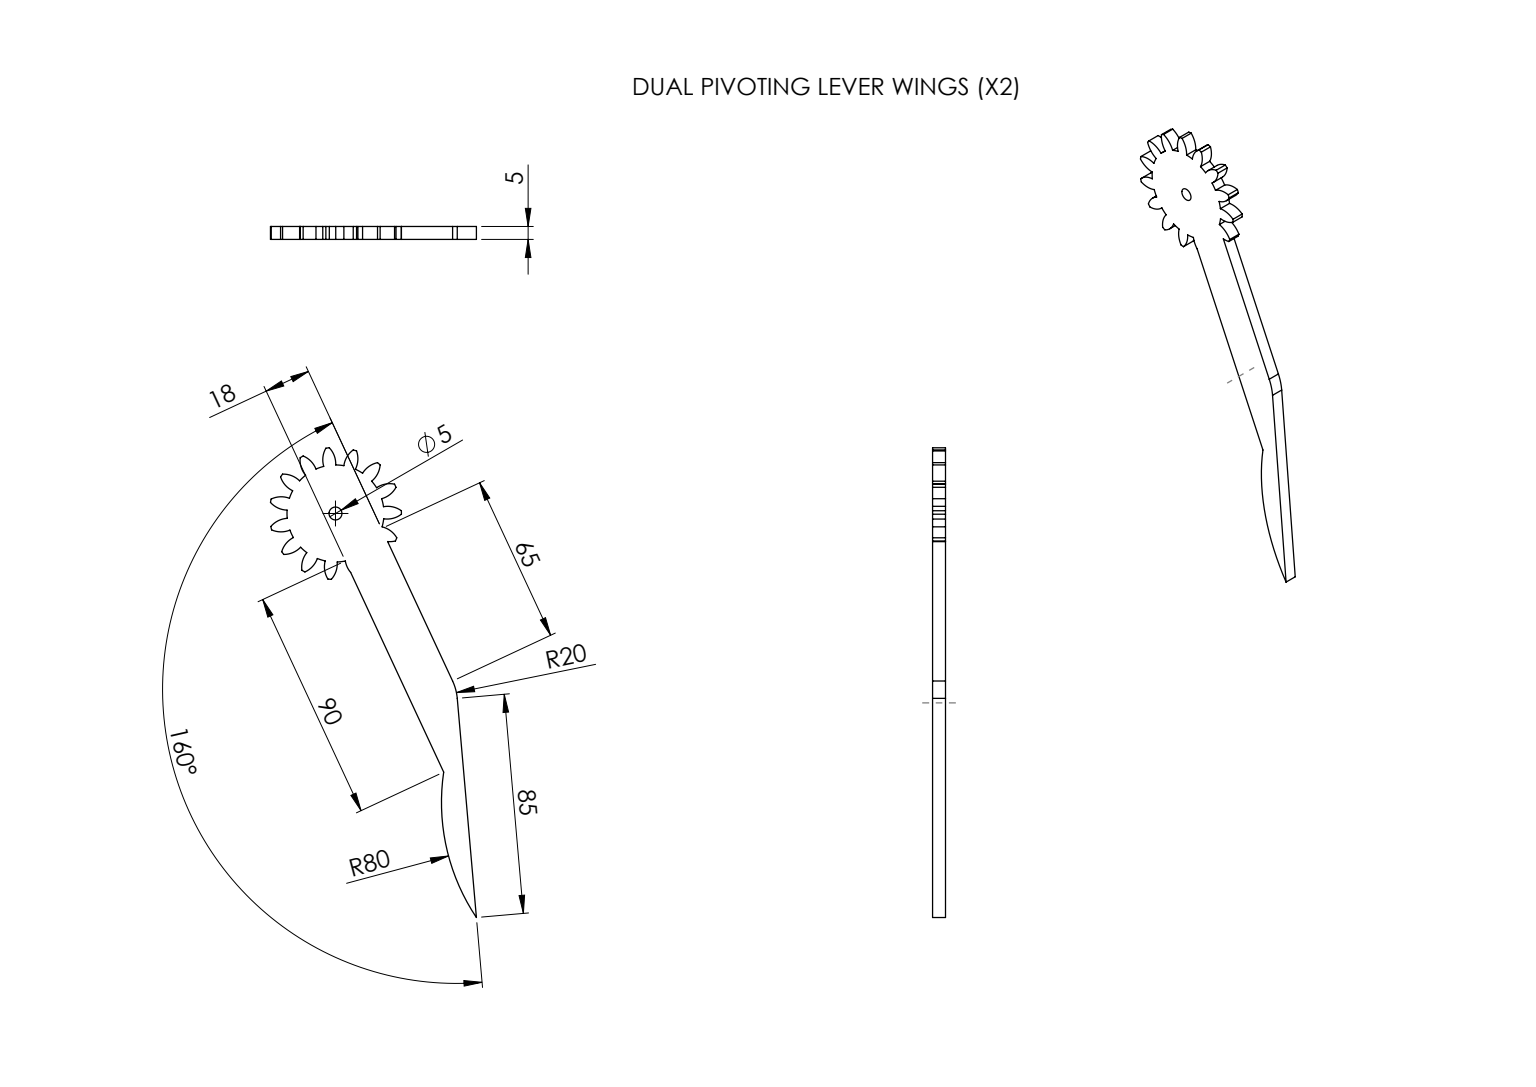
ISO-10303-21;
HEADER;
FILE_DESCRIPTION (('STEP AP214'),
    '1' );
FILE_NAME ('Dual Pivoting Lever Wings (x2).step',
    '2026-10-08T14:03:35',
    ( '' ),
    ( '' ),
    'SwSTEP 2.0',
    'SolidWorks 2026',
    '' );
FILE_SCHEMA (( 'AUTOMOTIVE_DESIGN' ));
ENDSEC;

DATA;
#2=ORIENTED_EDGE ( 'NONE', *, *, #10289, .F. ) ;
#4=VECTOR ( 'NONE', #10867, 1000.000000000000000 ) ;
#6=DIRECTION ( 'NONE',  ( 0.9960067511297464593, -0.08927794634716622324, 3.401418580343279473E-17 ) ) ;
#13=CARTESIAN_POINT ( 'NONE',  ( 34.99999999999958789, 1.104930248025249758E-13, -2.499999999999999112 ) ) ;
#17=EDGE_CURVE ( 'NONE', #9929, #10530, #4223, .T. ) ;
#25=EDGE_LOOP ( 'NONE', ( #11281, #8827, #8911, #8959 ) ) ;
#34=DIRECTION ( 'NONE',  ( 0.9960067511297463483, -0.08927794634716618161, 4.818676322152979407E-17 ) ) ;
#45=AXIS2_PLACEMENT_3D ( 'NONE', #8376, #5215, #8445 ) ;
#48=ORIENTED_EDGE ( 'NONE', *, *, #13831, .T. ) ;
#51=DIRECTION ( 'NONE',  ( 0.9960067511297463483, -0.08927794634716618161, 4.818676322152979407E-17 ) ) ;
#66=CARTESIAN_POINT ( 'NONE',  ( 34.99999999999958789, 1.104930248025249758E-13, -2.499999999999999112 ) ) ;
#68=DIRECTION ( 'NONE',  ( -6.158143864569485777E-17, -2.736152283717910599E-16, 1.000000000000000000 ) ) ;
#76=AXIS2_PLACEMENT_3D ( 'NONE', #13638, #11239, #6171 ) ;
#85=ORIENTED_EDGE ( 'NONE', *, *, #10554, .F. ) ;
#86=AXIS2_PLACEMENT_3D ( 'NONE', #6886, #3650, #3573 ) ;
#87=AXIS2_PLACEMENT_3D ( 'NONE', #13479, #2566, #7966 ) ;
#88=ADVANCED_FACE ( 'NONE', ( #12662 ), #10538, .T. ) ;
#89=DIRECTION ( 'NONE',  ( 6.158143864569485777E-17, 2.736152283717910599E-16, -1.000000000000000000 ) ) ;
#90=EDGE_CURVE ( 'NONE', #3108, #8314, #5574, .T. ) ;
#92=DIRECTION ( 'NONE',  ( -0.8735848310779960046, 0.4866719047884612293, 9.637352644305955116E-17 ) ) ;
#95=CARTESIAN_POINT ( 'NONE',  ( 21.12690199240172007, 12.61198448588842425, -2.499999999999996447 ) ) ;
#101=EDGE_CURVE ( 'NONE', #11832, #6555, #12065, .T. ) ;
#109=CARTESIAN_POINT ( 'NONE',  ( 43.14708730495711819, 24.16350488746832781, 2.500000000000007105 ) ) ;
#116=ORIENTED_EDGE ( 'NONE', *, *, #6600, .T. ) ;
#124=EDGE_CURVE ( 'NONE', #4194, #10453, #1869, .T. ) ;
#127=CYLINDRICAL_SURFACE ( 'NONE', #2611, 18.74900000001875000 ) ;
#128=CYLINDRICAL_SURFACE ( 'NONE', #1187, 18.74900000001875000 ) ;
#130=AXIS2_PLACEMENT_3D ( 'NONE', #4348, #7713, #2181 ) ;
#132=AXIS2_PLACEMENT_3D ( 'NONE', #2558, #4657, #7593 ) ;
#136=ORIENTED_EDGE ( 'NONE', *, *, #744, .F. ) ;
#153=CARTESIAN_POINT ( 'NONE',  ( 43.29712336220986657, 19.44704974301885159, -2.499999999999993783 ) ) ;
#155=( LENGTH_UNIT ( ) NAMED_UNIT ( * ) SI_UNIT ( .MILLI., .METRE. ) );
#157=DIRECTION ( 'NONE',  ( -0.6001121574638169642, 0.7999158696163758409, 1.927470528861191270E-16 ) ) ;
#160=CYLINDRICAL_SURFACE ( 'NONE', #3931, 25.50000000002549783 ) ;
#161=ORIENTED_EDGE ( 'NONE', *, *, #4188, .T. ) ;
#163=ORIENTED_EDGE ( 'NONE', *, *, #556, .F. ) ;
#167=ORIENTED_EDGE ( 'NONE', *, *, #10705, .F. ) ;
#168=CYLINDRICAL_SURFACE ( 'NONE', #12862, 25.50000000002549783 ) ;
#170=DIRECTION ( 'NONE',  ( -6.158143864569485777E-17, -2.736152283717910599E-16, 1.000000000000000000 ) ) ;
#172=CYLINDRICAL_SURFACE ( 'NONE', #13260, 80.00000000000001421 ) ;
#175=CARTESIAN_POINT ( 'NONE',  ( 53.63671053572210923, -2.048907369402451106, 2.500000000000000444 ) ) ;
#182=VERTEX_POINT ( 'NONE', #256 ) ;
#186=CARTESIAN_POINT ( 'NONE',  ( 41.86252833142972918, 24.55922850786694056, 2.500000000000007105 ) ) ;
#189=DIRECTION ( 'NONE',  ( -6.158143864569485777E-17, -2.736152283717910599E-16, 1.000000000000000000 ) ) ;
#197=ADVANCED_FACE ( 'NONE', ( #5497 ), #1357, .T. ) ;
#203=CARTESIAN_POINT ( 'NONE',  ( 80.29381926039658879, -64.72749139719506672, -2.500000000000000000 ) ) ;
#209=EDGE_LOOP ( 'NONE', ( #5485, #10650, #4189, #10104 ) ) ;
#216=ORIENTED_EDGE ( 'NONE', *, *, #1663, .T. ) ;
#220=DIRECTION ( 'NONE',  ( 0.1928999275155749149, 0.9812184353977894125, 2.775705599192072226E-16 ) ) ;
#222=DIRECTION ( 'NONE',  ( 6.158143864569485777E-17, 2.736152283717910599E-16, -1.000000000000000000 ) ) ;
#239=CIRCLE ( 'NONE', #906, 9.000000000008999024 ) ;
#242=ORIENTED_EDGE ( 'NONE', *, *, #7205, .T. ) ;
#254=CARTESIAN_POINT ( 'NONE',  ( 51.25836974494252019, 19.64472991003004054, 6.505213034913026604E-15 ) ) ;
#256=CARTESIAN_POINT ( 'NONE',  ( 23.90723890023449627, -15.11541108221136476, -2.500000000000003553 ) ) ;
#279=ORIENTED_EDGE ( 'NONE', *, *, #778, .T. ) ;
#288=FILL_AREA_STYLE_COLOUR ( '', #11871 ) ;
#290=DIRECTION ( 'NONE',  ( 0.000000000000000000, 0.000000000000000000, -1.000000000000000000 ) ) ;
#294=ORIENTED_EDGE ( 'NONE', *, *, #6674, .T. ) ;
#314=ORIENTED_EDGE ( 'NONE', *, *, #9696, .T. ) ;
#315=ORIENTED_EDGE ( 'NONE', *, *, #6674, .F. ) ;
#317=DIRECTION ( 'NONE',  ( -6.158143864569485777E-17, -2.736152283717910599E-16, 1.000000000000000000 ) ) ;
#319=CARTESIAN_POINT ( 'NONE',  ( 52.26118412238654543, 18.64354822589355365, 2.500000000000006217 ) ) ;
#321=EDGE_LOOP ( 'NONE', ( #4799, #6179, #1264, #10017 ) ) ;
#335=CARTESIAN_POINT ( 'NONE',  ( 14.79219767565757770, 6.218900627562692129, -2.499999999999999112 ) ) ;
#339=CIRCLE ( 'NONE', #9953, 18.74900000001874645 ) ;
#343=ORIENTED_EDGE ( 'NONE', *, *, #10693, .T. ) ;
#344=CARTESIAN_POINT ( 'NONE',  ( 22.31663499682298735, 16.91633092580596198, -2.499999999999995559 ) ) ;
#352=EDGE_CURVE ( 'NONE', #2949, #3802, #8059, .T. ) ;
#353=ORIENTED_EDGE ( 'NONE', *, *, #1966, .F. ) ;
#358=EDGE_LOOP ( 'NONE', ( #9572, #5128, #4628, #12509 ) ) ;
#361=CARTESIAN_POINT ( 'NONE',  ( 89.49979561504950709, -156.1132911148542917, 2.500000000000000000 ) ) ;
#363=DIRECTION ( 'NONE',  ( -6.158143864569485777E-17, -2.736152283717910599E-16, 1.000000000000000000 ) ) ;
#378=DIRECTION ( 'NONE',  ( -6.158143864569485777E-17, -2.736152283717910599E-16, 1.000000000000000000 ) ) ;
#382=DIRECTION ( 'NONE',  ( 1.000000000000000000, 0.000000000000000000, 0.000000000000000000 ) ) ;
#389=CARTESIAN_POINT ( 'NONE',  ( 37.49001687782395464, -0.2231948658678056807, 2.500000000000000000 ) ) ;
#390=DIRECTION ( 'NONE',  ( 0.9960067511297464593, -0.08927794634716622324, 3.401418580343279473E-17 ) ) ;
#391=CARTESIAN_POINT ( 'NONE',  ( 22.49448184590488609, 22.22300645049885048, 5.637851296924623057E-15 ) ) ;
#393=ORIENTED_EDGE ( 'NONE', *, *, #4024, .T. ) ;
#403=DIRECTION ( 'NONE',  ( 0.000000000000000000, 0.000000000000000000, 1.000000000000000000 ) ) ;
#404=CARTESIAN_POINT ( 'NONE',  ( 34.99999999999958789, 1.104930248025249758E-13, -2.499999999999999112 ) ) ;
#412=DIRECTION ( 'NONE',  ( 0.9960067511297463483, -0.08927794634716620936, 4.818676322152979407E-17 ) ) ;
#419=PLANE ( 'NONE',  #6579 ) ;
#420=VERTEX_POINT ( 'NONE', #8511 ) ;
#425=VERTEX_POINT ( 'NONE', #1859 ) ;
#434=DIRECTION ( 'NONE',  ( 0.9960067511297463483, -0.08927794634716620936, 4.626175998653454121E-17 ) ) ;
#439=ORIENTED_EDGE ( 'NONE', *, *, #8493, .T. ) ;
#442=AXIS2_PLACEMENT_3D ( 'NONE', #5645, #10070, #6772 ) ;
#445=EDGE_LOOP ( 'NONE', ( #13282, #343, #13733, #11306 ) ) ;
#456=EDGE_CURVE ( 'NONE', #10530, #1244, #10744, .T. ) ;
#458=EDGE_CURVE ( 'NONE', #11452, #4720, #10511, .T. ) ;
#460=ORIENTED_EDGE ( 'NONE', *, *, #2158, .F. ) ;
#468=ORIENTED_EDGE ( 'NONE', *, *, #11757, .F. ) ;
#469=DIRECTION ( 'NONE',  ( -6.158143864569485777E-17, -2.736152283717910599E-16, 1.000000000000000000 ) ) ;
#490=DIRECTION ( 'NONE',  ( -6.158143864569485777E-17, -2.736152283717910599E-16, 1.000000000000000000 ) ) ;
#508=CARTESIAN_POINT ( 'NONE',  ( 17.38503225228318883, -6.421675190136375555, 2.499999999999996891 ) ) ;
#517=EDGE_CURVE ( 'NONE', #3335, #6792, #6412, .T. ) ;
#520=ORIENTED_EDGE ( 'NONE', *, *, #4473, .T. ) ;
#526=CARTESIAN_POINT ( 'NONE',  ( 34.99999999999958789, 1.104930248025249758E-13, -2.499999999999999112 ) ) ;
#530=CARTESIAN_POINT ( 'NONE',  ( 19.06870874253413461, 13.90050210118286245, -2.499999999999996447 ) ) ;
#534=VERTEX_POINT ( 'NONE', #109 ) ;
#544=CARTESIAN_POINT ( 'NONE',  ( 52.82363224725100537, -5.817485239812894449, 2.500000000000000000 ) ) ;
#556=EDGE_CURVE ( 'NONE', #5704, #4432, #4456, .T. ) ;
#566=DIRECTION ( 'NONE',  ( 0.9960067511297464593, -0.08927794634716622324, 3.401418580343279473E-17 ) ) ;
#576=VERTEX_POINT ( 'NONE', #10197 ) ;
#586=VECTOR ( 'NONE', #4081, 1000.000000000000000 ) ;
#608=ORIENTED_EDGE ( 'NONE', *, *, #9776, .F. ) ;
#609=CARTESIAN_POINT ( 'NONE',  ( 34.99999999999958789, 1.104930248025249758E-13, -2.499999999999999112 ) ) ;
#614=EDGE_CURVE ( 'NONE', #8676, #13485, #6969, .T. ) ;
#617=DIRECTION ( 'NONE',  ( 0.000000000000000000, 0.000000000000000000, -1.000000000000000000 ) ) ;
#646=ADVANCED_FACE ( 'NONE', ( #3590 ), #7879, .T. ) ;
#656=CARTESIAN_POINT ( 'NONE',  ( 47.16901142695026294, 17.29003067336574517, -2.499999999999993783 ) ) ;
#658=CYLINDRICAL_SURFACE ( 'NONE', #13126, 25.50000000002549783 ) ;
#671=VECTOR ( 'NONE', #4287, 1000.000000000000000 ) ;
#674=DIRECTION ( 'NONE',  ( -6.158143864569485777E-17, -2.736152283717910599E-16, 1.000000000000000000 ) ) ;
#682=ORIENTED_EDGE ( 'NONE', *, *, #7351, .F. ) ;
#686=EDGE_CURVE ( 'NONE', #4911, #5054, #12997, .T. ) ;
#687=AXIS2_PLACEMENT_3D ( 'NONE', #7573, #11991, #11787 ) ;
#704=EDGE_CURVE ( 'NONE', #3094, #2145, #2456, .T. ) ;
#706=AXIS2_PLACEMENT_3D ( 'NONE', #5977, #6041, #11432 ) ;
#708=EDGE_CURVE ( 'NONE', #4432, #2174, #1790, .T. ) ;
#720=DIRECTION ( 'NONE',  ( -6.158143864569485777E-17, -2.736152283717910599E-16, 1.000000000000000000 ) ) ;
#723=EDGE_CURVE ( 'NONE', #5202, #2631, #4244, .T. ) ;
#725=EDGE_CURVE ( 'NONE', #6555, #9666, #3819, .T. ) ;
#730=CYLINDRICAL_SURFACE ( 'NONE', #10911, 9.000000000008999024 ) ;
#731=CARTESIAN_POINT ( 'NONE',  ( 58.17953216333035726, -10.62823074130461620, -8.673617379884035472E-16 ) ) ;
#735=DIRECTION ( 'NONE',  ( -1.000000000000000000, 0.000000000000000000, 0.000000000000000000 ) ) ;
#736=ORIENTED_EDGE ( 'NONE', *, *, #8755, .F. ) ;
#740=DIRECTION ( 'NONE',  ( 6.158143864569485777E-17, 2.736152283717910599E-16, -1.000000000000000000 ) ) ;
#744=EDGE_CURVE ( 'NONE', #12212, #7540, #11649, .T. ) ;
#750=VERTEX_POINT ( 'NONE', #1329 ) ;
#752=VERTEX_POINT ( 'NONE', #11007 ) ;
#756=ORIENTED_EDGE ( 'NONE', *, *, #708, .T. ) ;
#771=DIRECTION ( 'NONE',  ( -6.158143864569485777E-17, -2.736152283717910599E-16, 1.000000000000000000 ) ) ;
#775=CARTESIAN_POINT ( 'NONE',  ( 53.63671053572210923, -2.048907369402450218, -2.499999999999998224 ) ) ;
#778=EDGE_CURVE ( 'NONE', #3832, #2373, #7776, .T. ) ;
#785=VECTOR ( 'NONE', #10919, 1000.000000000000227 ) ;
#788=DIRECTION ( 'NONE',  ( -6.158143864569485777E-17, -2.736152283717910599E-16, 1.000000000000000000 ) ) ;
#789=DIRECTION ( 'NONE',  ( -6.158143864569485777E-17, -2.736152283717910599E-16, 1.000000000000000000 ) ) ;
#791=DIRECTION ( 'NONE',  ( -6.158143864569485777E-17, -2.736152283717910599E-16, 1.000000000000000000 ) ) ;
#796=EDGE_CURVE ( 'NONE', #2373, #4518, #239, .T. ) ;
#800=ORIENTED_EDGE ( 'NONE', *, *, #1340, .F. ) ;
#804=CARTESIAN_POINT ( 'NONE',  ( 34.99999999999958789, 1.091249486606660213E-13, 2.500000000000000000 ) ) ;
#811=CARTESIAN_POINT ( 'NONE',  ( 27.45605056404223987, 17.16431845161426040, -2.499999999999994671 ) ) ;
#815=AXIS2_PLACEMENT_3D ( 'NONE', #10025, #10171, #5821 ) ;
#818=CARTESIAN_POINT ( 'NONE',  ( 16.34455450841068469, -1.870656171256066758, 2.499999999999998224 ) ) ;
#822=VECTOR ( 'NONE', #5012, 1000.000000000000000 ) ;
#824=LINE ( 'NONE', #6347, #9737 ) ;
#825=ORIENTED_EDGE ( 'NONE', *, *, #8248, .F. ) ;
#829=CIRCLE ( 'NONE', #87, 20.00000000000001066 ) ;
#838=ORIENTED_EDGE ( 'NONE', *, *, #9996, .T. ) ;
#844=DIRECTION ( 'NONE',  ( -6.158143864569485777E-17, -2.736152283717910599E-16, 1.000000000000000000 ) ) ;
#848=DIRECTION ( 'NONE',  ( -6.158143864569485777E-17, -2.736152283717910599E-16, 1.000000000000000000 ) ) ;
#851=LINE ( 'NONE', #5055, #5935 ) ;
#856=CARTESIAN_POINT ( 'NONE',  ( 32.50998312217522113, 0.2231948658680386610, -47.50005079999998969 ) ) ;
#857=CARTESIAN_POINT ( 'NONE',  ( 82.09155748149851206, -71.43674177705591433, -2.500000000000000000 ) ) ;
#858=DIRECTION ( 'NONE',  ( -6.158143864569485777E-17, -2.736152283717910599E-16, 1.000000000000000000 ) ) ;
#864=VECTOR ( 'NONE', #910, 1000.000000000000000 ) ;
#881=DIRECTION ( 'NONE',  ( 0.9960067511297463483, -0.08927794634716620936, 4.818676322152979407E-17 ) ) ;
#899=ORIENTED_EDGE ( 'NONE', *, *, #12455, .T. ) ;
#906=AXIS2_PLACEMENT_3D ( 'NONE', #5832, #13522, #6046 ) ;
#910=DIRECTION ( 'NONE',  ( -6.158143864569485777E-17, -2.736152283717910599E-16, 1.000000000000000000 ) ) ;
#917=EDGE_LOOP ( 'NONE', ( #12551, #1766, #7020, #2213 ) ) ;
#922=ORIENTED_EDGE ( 'NONE', *, *, #12535, .F. ) ;
#925=DIRECTION ( 'NONE',  ( 0.1928999275155751925, 0.9812184353977893014, 2.891205793291787151E-16 ) ) ;
#926=CARTESIAN_POINT ( 'NONE',  ( 13.94188849117746010, 1.893657697999892475, 2.499999999999999112 ) ) ;
#928=CARTESIAN_POINT ( 'NONE',  ( 22.49448184590488609, 22.22300645049884693, -2.499999999999993783 ) ) ;
#929=DIRECTION ( 'NONE',  ( 0.000000000000000000, 0.000000000000000000, -1.000000000000000000 ) ) ;
#930=AXIS2_PLACEMENT_3D ( 'NONE', #2671, #4852, #1475 ) ;
#945=LINE ( 'NONE', #811, #6925 ) ;
#946=CARTESIAN_POINT ( 'NONE',  ( 26.69171018101576465, -19.44228176112429551, -2.500000000000004441 ) ) ;
#956=EDGE_LOOP ( 'NONE', ( #10577, #10149, #7801, #1791 ) ) ;
#970=EDGE_CURVE ( 'NONE', #11470, #1977, #6576, .T. ) ;
#971=AXIS2_PLACEMENT_3D ( 'NONE', #3341, #7616, #566 ) ;
#988=VERTEX_POINT ( 'NONE', #13058 ) ;
#992=DIRECTION ( 'NONE',  ( 6.158143864569485777E-17, 2.736152283717910599E-16, -1.000000000000000000 ) ) ;
#994=LINE ( 'NONE', #857, #4463 ) ;
#999=ORIENTED_EDGE ( 'NONE', *, *, #11843, .F. ) ;
#1007=DIRECTION ( 'NONE',  ( -0.9960067511297463483, 0.08927794634716618161, -4.818676322152979407E-17 ) ) ;
#1009=DIRECTION ( 'NONE',  ( -0.9960067511297463483, 0.08927794634716619548, 0.000000000000000000 ) ) ;
#1019=CARTESIAN_POINT ( 'NONE',  ( 47.69307742500824787, -16.90904448151677286, -2.500000000000002665 ) ) ;
#1023=LINE ( 'NONE', #5290, #2346 ) ;
#1024=AXIS2_PLACEMENT_3D ( 'NONE', #3165, #1075, #2972 ) ;
#1025=EDGE_LOOP ( 'NONE', ( #2026, #393, #13216, #12913 ) ) ;
#1037=AXIS2_PLACEMENT_3D ( 'NONE', #4299, #2123, #12878 ) ;
#1049=DIRECTION ( 'NONE',  ( -6.158143864569485777E-17, -2.736152283717910599E-16, 1.000000000000000000 ) ) ;
#1055=EDGE_LOOP ( 'NONE', ( #5377, #10230, #6043, #5850 ) ) ;
#1056=DIRECTION ( 'NONE',  ( -6.158143864569485777E-17, -2.736152283717910599E-16, 1.000000000000000000 ) ) ;
#1057=ORIENTED_EDGE ( 'NONE', *, *, #1663, .F. ) ;
#1062=FACE_OUTER_BOUND ( 'NONE', #5350, .T. ) ;
#1074=ORIENTED_EDGE ( 'NONE', *, *, #3879, .T. ) ;
#1075=DIRECTION ( 'NONE',  ( -6.158143864569485777E-17, -2.736152283717910599E-16, 1.000000000000000000 ) ) ;
#1096=FACE_OUTER_BOUND ( 'NONE', #7554, .T. ) ;
#1100=CARTESIAN_POINT ( 'NONE',  ( 14.20591609908153430, -14.75994833063034406, -2.500000000000004441 ) ) ;
#1106=AXIS2_PLACEMENT_3D ( 'NONE', #4084, #6068, #10604 ) ;
#1108=CARTESIAN_POINT ( 'NONE',  ( 34.99999999999958789, 1.104930248025249758E-13, -2.499999999999999112 ) ) ;
#1110=AXIS2_PLACEMENT_3D ( 'NONE', #13074, #1328, #3491 ) ;
#1118=EDGE_CURVE ( 'NONE', #2729, #11470, #9632, .T. ) ;
#1119=ORIENTED_EDGE ( 'NONE', *, *, #6804, .F. ) ;
#1130=( NAMED_UNIT ( * ) SI_UNIT ( $, .STERADIAN. ) SOLID_ANGLE_UNIT ( ) );
#1144=CIRCLE ( 'NONE', #8981, 25.50000000002549783 ) ;
#1147=CARTESIAN_POINT ( 'NONE',  ( 34.99999999999958789, 1.104930248025249758E-13, -2.499999999999999112 ) ) ;
#1153=CARTESIAN_POINT ( 'NONE',  ( 50.89489709276795537, 9.943703908052052398, -2.499999999999994671 ) ) ;
#1157=DIRECTION ( 'NONE',  ( -6.158143864569485777E-17, -2.736152283717910599E-16, 1.000000000000000000 ) ) ;
#1163=CARTESIAN_POINT ( 'NONE',  ( 14.00979921278056040, -2.538005261501627086, -2.500000000000000888 ) ) ;
#1165=DIRECTION ( 'NONE',  ( -6.158143864569485777E-17, -2.736152283717910599E-16, 1.000000000000000000 ) ) ;
#1168=DIRECTION ( 'NONE',  ( 0.9960067511297463483, -0.08927794634716620936, 4.626175998653454121E-17 ) ) ;
#1174=DIRECTION ( 'NONE',  ( -0.2228746399763467390, 0.9748471135800802490, 2.409338161076489210E-16 ) ) ;
#1177=SURFACE_STYLE_FILL_AREA ( #6501 ) ;
#1178=VERTEX_POINT ( 'NONE', #4654 ) ;
#1180=DIRECTION ( 'NONE',  ( 0.9960067511297463483, -0.08927794634716620936, 4.626175998653454121E-17 ) ) ;
#1187=AXIS2_PLACEMENT_3D ( 'NONE', #3327, #7602, #3393 ) ;
#1198=FACE_OUTER_BOUND ( 'NONE', #4757, .T. ) ;
#1206=CARTESIAN_POINT ( 'NONE',  ( 35.65577094119244350, -20.24578327824959345, -2.500000000000003997 ) ) ;
#1211=CARTESIAN_POINT ( 'NONE',  ( 43.14708730495711819, 24.16350488746832781, 7.806255641895631925E-15 ) ) ;
#1219=EDGE_CURVE ( 'NONE', #3278, #2483, #11318, .T. ) ;
#1221=CARTESIAN_POINT ( 'NONE',  ( 35.08961652778860696, 18.74878582411816197, -2.499999999999993783 ) ) ;
#1224=FACE_OUTER_BOUND ( 'NONE', #917, .T. ) ;
#1243=ORIENTED_EDGE ( 'NONE', *, *, #7794, .F. ) ;
#1244=VERTEX_POINT ( 'NONE', #1713 ) ;
#1246=AXIS2_PLACEMENT_3D ( 'NONE', #4641, #1628, #9135 ) ;
#1247=DIRECTION ( 'NONE',  ( 6.158143864569485777E-17, 2.736152283717910599E-16, -1.000000000000000000 ) ) ;
#1248=DIRECTION ( 'NONE',  ( 0.4206864060305147146, -0.9072061219927525233, -2.409338161076489703E-16 ) ) ;
#1250=VECTOR ( 'NONE', #11018, 1000.000000000000000 ) ;
#1257=VERTEX_POINT ( 'NONE', #3812 ) ;
#1264=ORIENTED_EDGE ( 'NONE', *, *, #10289, .T. ) ;
#1269=DIRECTION ( 'NONE',  ( 0.4226182617407009401, -0.9063077870366491595, -0.000000000000000000 ) ) ;
#1271=FACE_OUTER_BOUND ( 'NONE', #11973, .T. ) ;
#1272=CARTESIAN_POINT ( 'NONE',  ( 21.51985683731163945, -13.03114504999992995, -2.500000000000004441 ) ) ;
#1279=EDGE_CURVE ( 'NONE', #12858, #420, #13718, .T. ) ;
#1282=ORIENTED_EDGE ( 'NONE', *, *, #6005, .F. ) ;
#1290=ORIENTED_EDGE ( 'NONE', *, *, #4117, .T. ) ;
#1291=EDGE_CURVE ( 'NONE', #7693, #12930, #4483, .T. ) ;
#1311=DIRECTION ( 'NONE',  ( 6.158143864569485777E-17, 2.736152283717910599E-16, -1.000000000000000000 ) ) ;
#1322=DIRECTION ( 'NONE',  ( 0.9960067511297464593, -0.08927794634716622324, 3.401418580343279473E-17 ) ) ;
#1327=VECTOR ( 'NONE', #9078, 1000.000000000000000 ) ;
#1328=DIRECTION ( 'NONE',  ( -6.158143864569485777E-17, -2.736152283717910599E-16, 1.000000000000000000 ) ) ;
#1329=CARTESIAN_POINT ( 'NONE',  ( 40.87368016229836343, -22.78235879061915625, 2.499999999999993783 ) ) ;
#1336=CARTESIAN_POINT ( 'NONE',  ( 34.99999999999958789, 1.091249486606660213E-13, 2.500000000000000000 ) ) ;
#1340=EDGE_CURVE ( 'NONE', #6463, #2032, #1803, .T. ) ;
#1344=ORIENTED_EDGE ( 'NONE', *, *, #970, .T. ) ;
#1353=EDGE_LOOP ( 'NONE', ( #10331, #161, #8745, #6168 ) ) ;
#1357=CYLINDRICAL_SURFACE ( 'NONE', #12995, 18.74900000001875000 ) ;
#1368=AXIS2_PLACEMENT_3D ( 'NONE', #5270, #9352, #4013 ) ;
#1374=FACE_OUTER_BOUND ( 'NONE', #10512, .T. ) ;
#1377=ORIENTED_EDGE ( 'NONE', *, *, #1772, .T. ) ;
#1378=CYLINDRICAL_SURFACE ( 'NONE', #10821, 9.000000000008999024 ) ;
#1384=ADVANCED_FACE ( 'NONE', ( #9399 ), #12637, .T. ) ;
#1389=ORIENTED_EDGE ( 'NONE', *, *, #4269, .F. ) ;
#1393=CARTESIAN_POINT ( 'NONE',  ( 34.99999999999958789, 1.063887963769481123E-13, 12.50000000000000000 ) ) ;
#1395=CARTESIAN_POINT ( 'NONE',  ( 43.63403238902020576, 20.33700654369049587, -2.499999999999992895 ) ) ;
#1397=CARTESIAN_POINT ( 'NONE',  ( 43.29712336220986657, 19.44704974301885159, 2.500000000000005773 ) ) ;
#1401=EDGE_CURVE ( 'NONE', #4911, #12400, #10094, .T. ) ;
#1406=CARTESIAN_POINT ( 'NONE',  ( 155.9864723944028810, -111.6214737678657087, 2.500000000000000000 ) ) ;
#1409=CARTESIAN_POINT ( 'NONE',  ( 0.000000000000000000, 0.000000000000000000, 0.000000000000000000 ) ) ;
#1429=ORIENTED_EDGE ( 'NONE', *, *, #9258, .T. ) ;
#1455=ORIENTED_EDGE ( 'NONE', *, *, #6677, .F. ) ;
#1463=EDGE_CURVE ( 'NONE', #9210, #11257, #4951, .T. ) ;
#1467=CARTESIAN_POINT ( 'NONE',  ( 34.99999999999958789, 1.104930248025249758E-13, -2.499999999999999112 ) ) ;
#1469=CARTESIAN_POINT ( 'NONE',  ( 32.05482125692310547, -25.32934902781011743, -6.505213034913026604E-15 ) ) ;
#1470=CARTESIAN_POINT ( 'NONE',  ( 22.84091969677297485, -17.29701610032388359, -2.500000000000004441 ) ) ;
#1473=VERTEX_POINT ( 'NONE', #13266 ) ;
#1474=MECHANICAL_DESIGN_GEOMETRIC_PRESENTATION_REPRESENTATION('',(#5507),#12915);
#1475=DIRECTION ( 'NONE',  ( 0.9960067511297464593, -0.08927794634716622324, 3.401418580343279473E-17 ) ) ;
#1481=CARTESIAN_POINT ( 'NONE',  ( 55.99165482216006495, 2.525950835318802934, 2.500000000000002220 ) ) ;
#1482=ADVANCED_FACE ( 'NONE', ( #3900 ), #7121, .T. ) ;
#1494=ORIENTED_EDGE ( 'NONE', *, *, #725, .F. ) ;
#1504=LINE ( 'NONE', #4249, #11680 ) ;
#1513=CIRCLE ( 'NONE', #5438, 25.50000000002549783 ) ;
#1535=AXIS2_PLACEMENT_3D ( 'NONE', #11860, #12937, #4416 ) ;
#1538=EDGE_CURVE ( 'NONE', #11754, #750, #7410, .T. ) ;
#1541=ORIENTED_EDGE ( 'NONE', *, *, #4175, .T. ) ;
#1548=EDGE_LOOP ( 'NONE', ( #2270, #11697, #4778, #6657 ) ) ;
#1552=FACE_OUTER_BOUND ( 'NONE', #10987, .T. ) ;
#1556=DIRECTION ( 'NONE',  ( -6.158143864569485777E-17, -2.736152283717910599E-16, 1.000000000000000000 ) ) ;
#1561=CARTESIAN_POINT ( 'NONE',  ( 14.79219767565757770, 6.218900627562692129, -2.499999999999999112 ) ) ;
#1564=EDGE_CURVE ( 'NONE', #4257, #11572, #2193, .T. ) ;
#1568=AXIS2_PLACEMENT_3D ( 'NONE', #4156, #7447, #8306 ) ;
#1569=DIRECTION ( 'NONE',  ( -0.08715574274765883200, 0.9961946980917454342, 0.000000000000000000 ) ) ;
#1574=LINE ( 'NONE', #1776, #7953 ) ;
#1581=DIRECTION ( 'NONE',  ( -6.158143864569485777E-17, -2.736152283717910599E-16, 1.000000000000000000 ) ) ;
#1582=PLANE ( 'NONE',  #2090 ) ;
#1584=CYLINDRICAL_SURFACE ( 'NONE', #5114, 9.000000000008999024 ) ;
#1585=ADVANCED_FACE ( 'NONE', ( #6678 ), #13166, .T. ) ;
#1606=AXIS2_PLACEMENT_3D ( 'NONE', #6003, #7042, #13605 ) ;
#1607=CARTESIAN_POINT ( 'NONE',  ( 34.99999999999958789, 1.091249486606660213E-13, 2.500000000000000000 ) ) ;
#1608=EDGE_LOOP ( 'NONE', ( #6442, #1785, #12436, #12671 ) ) ;
#1611=CARTESIAN_POINT ( 'NONE',  ( 37.49001687782395464, -0.2231948658678050423, -2.499999999999997335 ) ) ;
#1616=ORIENTED_EDGE ( 'NONE', *, *, #13052, .F. ) ;
#1628=DIRECTION ( 'NONE',  ( -6.158143864569485777E-17, -2.736152283717910599E-16, 1.000000000000000000 ) ) ;
#1632=EDGE_LOOP ( 'NONE', ( #12045, #10879, #4615, #10703 ) ) ;
#1642=EDGE_CURVE ( 'NONE', #4432, #9210, #11254, .T. ) ;
#1645=AXIS2_PLACEMENT_3D ( 'NONE', #6464, #9685, #92 ) ;
#1652=EDGE_CURVE ( 'NONE', #9058, #2729, #2495, .T. ) ;
#1656=CARTESIAN_POINT ( 'NONE',  ( 38.24615002434714484, 18.46584715143433542, 2.500000000000005329 ) ) ;
#1659=VERTEX_POINT ( 'NONE', #7367 ) ;
#1661=DIRECTION ( 'NONE',  ( 0.9960067511297464593, -0.08927794634716622324, 6.802837160686558945E-17 ) ) ;
#1663=EDGE_CURVE ( 'NONE', #3310, #9058, #3592, .T. ) ;
#1664=ORIENTED_EDGE ( 'NONE', *, *, #3879, .F. ) ;
#1683=VECTOR ( 'NONE', #7325, 1000.000000000000000 ) ;
#1689=VECTOR ( 'NONE', #4035, 1000.000000000000000 ) ;
#1697=DIRECTION ( 'NONE',  ( 0.01532218268402011502, -0.9998826084685129567, -2.891205793291787644E-16 ) ) ;
#1700=CARTESIAN_POINT ( 'NONE',  ( 14.20591609908152009, -14.75994833063034761, 2.499999999999994671 ) ) ;
#1711=AXIS2_PLACEMENT_3D ( 'NONE', #10520, #8355, #6123 ) ;
#1713=CARTESIAN_POINT ( 'NONE',  ( 35.08961652778860696, 18.74878582411816197, 2.500000000000005329 ) ) ;
#1719=CARTESIAN_POINT ( 'NONE',  ( 17.19653809941365452, 5.878923826270381348, -2.499999999999999112 ) ) ;
#1720=CYLINDRICAL_SURFACE ( 'NONE', #8580, 9.000000000008999024 ) ;
#1723=FACE_OUTER_BOUND ( 'NONE', #3899, .T. ) ;
#1724=EDGE_CURVE ( 'NONE', #7206, #13532, #6973, .T. ) ;
#1728=DIRECTION ( 'NONE',  ( -6.158143864569485777E-17, -2.736152283717910599E-16, 1.000000000000000000 ) ) ;
#1736=CARTESIAN_POINT ( 'NONE',  ( 37.49001687782395464, -0.2231948658677927189, -47.50005079999998969 ) ) ;
#1737=CARTESIAN_POINT ( 'NONE',  ( 34.66997162884352690, 21.14050806081579736, 2.500000000000005773 ) ) ;
#1740=ORIENTED_EDGE ( 'NONE', *, *, #8641, .T. ) ;
#1751=DIRECTION ( 'NONE',  ( -6.158143864569485777E-17, -2.736152283717910599E-16, 1.000000000000000000 ) ) ;
#1752=AXIS2_PLACEMENT_3D ( 'NONE', #13, #7158, #2038 ) ;
#1753=VERTEX_POINT ( 'NONE', #3704 ) ;
#1756=CIRCLE ( 'NONE', #9593, 25.50000000002549783 ) ;
#1766=ORIENTED_EDGE ( 'NONE', *, *, #8130, .F. ) ;
#1770=DIRECTION ( 'NONE',  ( -6.158143864569485777E-17, -2.736152283717910599E-16, 1.000000000000000000 ) ) ;
#1771=ORIENTED_EDGE ( 'NONE', *, *, #11775, .F. ) ;
#1772=EDGE_CURVE ( 'NONE', #12816, #4304, #9219, .T. ) ;
#1776=CARTESIAN_POINT ( 'NONE',  ( 27.98552063842490867, -17.38741154648219833, -2.500000000000004441 ) ) ;
#1777=CIRCLE ( 'NONE', #7363, 25.50000000002549783 ) ;
#1785=ORIENTED_EDGE ( 'NONE', *, *, #556, .T. ) ;
#1790=CIRCLE ( 'NONE', #12787, 18.74900000001875000 ) ;
#1791=ORIENTED_EDGE ( 'NONE', *, *, #7351, .T. ) ;
#1802=LINE ( 'NONE', #6355, #10592 ) ;
#1803=CIRCLE ( 'NONE', #12345, 9.000000000009002576 ) ;
#1804=CARTESIAN_POINT ( 'NONE',  ( 18.44105126153190710, 8.793532718851094998, -2.499999999999998224 ) ) ;
#1816=EDGE_CURVE ( 'NONE', #7931, #7120, #9441, .T. ) ;
#1819=CARTESIAN_POINT ( 'NONE',  ( 35.66405164569891184, -18.73723662690267133, 2.499999999999994671 ) ) ;
#1827=CARTESIAN_POINT ( 'NONE',  ( 43.29712336220986657, 19.44704974301885159, -2.499999999999993783 ) ) ;
#1835=AXIS2_PLACEMENT_3D ( 'NONE', #3086, #5122, #7355 ) ;
#1842=ORIENTED_EDGE ( 'NONE', *, *, #11330, .T. ) ;
#1845=DIRECTION ( 'NONE',  ( -6.158143864569485777E-17, -2.736152283717910599E-16, 1.000000000000000000 ) ) ;
#1848=DIRECTION ( 'NONE',  ( -0.4226182617407014397, 0.9063077870366489375, 0.000000000000000000 ) ) ;
#1859=CARTESIAN_POINT ( 'NONE',  ( 22.49448184590488609, 22.22300645049885048, 2.500000000000005329 ) ) ;
#1860=ORIENTED_EDGE ( 'NONE', *, *, #3852, .T. ) ;
#1865=EDGE_LOOP ( 'NONE', ( #7834, #6382, #7851, #1377 ) ) ;
#1869=LINE ( 'NONE', #12679, #11839 ) ;
#1878=ORIENTED_EDGE ( 'NONE', *, *, #90, .F. ) ;
#1892=ORIENTED_EDGE ( 'NONE', *, *, #8431, .T. ) ;
#1900=ORIENTED_EDGE ( 'NONE', *, *, #7122, .F. ) ;
#1902=DIRECTION ( 'NONE',  ( -6.158143864569485777E-17, -2.736152283717910599E-16, 1.000000000000000000 ) ) ;
#1906=CARTESIAN_POINT ( 'NONE',  ( 34.99999999999958789, 1.104930248025249758E-13, -2.499999999999999112 ) ) ;
#1915=CARTESIAN_POINT ( 'NONE',  ( 55.20422767451771051, -6.230504303137472277, 2.499999999999999556 ) ) ;
#1940=DIRECTION ( 'NONE',  ( -6.158143864569485777E-17, -2.736152283717910599E-16, 1.000000000000000000 ) ) ;
#1945=CARTESIAN_POINT ( 'NONE',  ( 155.9864723944028810, -111.6214737678657087, 2.500000000000000000 ) ) ;
#1965=DIRECTION ( 'NONE',  ( 0.9960067511297463483, -0.08927794634716618161, 4.818676322152979407E-17 ) ) ;
#1966=EDGE_CURVE ( 'NONE', #4027, #1473, #4698, .T. ) ;
#1977=VERTEX_POINT ( 'NONE', #12789 ) ;
#1978=ORIENTED_EDGE ( 'NONE', *, *, #11261, .F. ) ;
#1979=CIRCLE ( 'NONE', #3770, 9.000000000009002576 ) ;
#1981=DIRECTION ( 'NONE',  ( -6.158143864569485777E-17, -2.736152283717910599E-16, 1.000000000000000000 ) ) ;
#1984=EDGE_CURVE ( 'NONE', #4263, #6792, #13709, .T. ) ;
#1991=DIRECTION ( 'NONE',  ( 0.9960067511297464593, -0.08927794634716622324, 3.401418580343279473E-17 ) ) ;
#1992=ADVANCED_FACE ( 'NONE', ( #5131, #8295 ), #4146, .F. ) ;
#1999=EDGE_LOOP ( 'NONE', ( #12155, #9038, #1616, #5906 ) ) ;
#2012=VECTOR ( 'NONE', #7587, 1000.000000000000000 ) ;
#2026=ORIENTED_EDGE ( 'NONE', *, *, #970, .F. ) ;
#2029=AXIS2_PLACEMENT_3D ( 'NONE', #1827, #848, #9470 ) ;
#2032=VERTEX_POINT ( 'NONE', #6631 ) ;
#2033=ORIENTED_EDGE ( 'NONE', *, *, #1219, .T. ) ;
#2038=DIRECTION ( 'NONE',  ( 0.9960067511297464593, -0.08927794634716622324, 3.401418580343279473E-17 ) ) ;
#2080=VECTOR ( 'NONE', #10962, 1000.000000000000000 ) ;
#2081=ORIENTED_EDGE ( 'NONE', *, *, #13499, .T. ) ;
#2090=AXIS2_PLACEMENT_3D ( 'NONE', #5938, #617, #13545 ) ;
#2093=CARTESIAN_POINT ( 'NONE',  ( 53.14943414785363984, 10.84564612680554063, 2.500000000000003997 ) ) ;
#2123=DIRECTION ( 'NONE',  ( -6.158143864569485777E-17, -2.736152283717910599E-16, 1.000000000000000000 ) ) ;
#2124=ORIENTED_EDGE ( 'NONE', *, *, #1564, .F. ) ;
#2127=EDGE_LOOP ( 'NONE', ( #13732, #12195, #9992, #12842 ) ) ;
#2132=DIRECTION ( 'NONE',  ( 0.9960067511297464593, -0.08927794634716622324, 6.802837160686558945E-17 ) ) ;
#2142=ADVANCED_FACE ( 'NONE', ( #5088 ), #6477, .T. ) ;
#2145=VERTEX_POINT ( 'NONE', #818 ) ;
#2156=ADVANCED_FACE ( 'NONE', ( #13748 ), #4093, .T. ) ;
#2158=EDGE_CURVE ( 'NONE', #1257, #12816, #6610, .T. ) ;
#2164=CARTESIAN_POINT ( 'NONE',  ( 58.17953216333035726, -10.62823074130461265, -2.500000000000000888 ) ) ;
#2173=EDGE_CURVE ( 'NONE', #12949, #1257, #2227, .T. ) ;
#2174=VERTEX_POINT ( 'NONE', #5483 ) ;
#2177=DIRECTION ( 'NONE',  ( -0.9960067511297463483, 0.08927794634716618161, -4.818676322152979407E-17 ) ) ;
#2178=ORIENTED_EDGE ( 'NONE', *, *, #13534, .F. ) ;
#2181=DIRECTION ( 'NONE',  ( 0.9960067511297463483, -0.08927794634716618161, 4.818676322152979407E-17 ) ) ;
#2187=DIRECTION ( 'NONE',  ( -6.158143864569485777E-17, -2.736152283717910599E-16, 1.000000000000000000 ) ) ;
#2192=EDGE_LOOP ( 'NONE', ( #13564, #3313, #4409, #922 ) ) ;
#2193=LINE ( 'NONE', #8709, #8532 ) ;
#2213=ORIENTED_EDGE ( 'NONE', *, *, #12483, .T. ) ;
#2227=CIRCLE ( 'NONE', #11455, 9.000000000008999024 ) ;
#2230=CARTESIAN_POINT ( 'NONE',  ( 10.11726280447958182, 5.576682675210010487, 4.336808689942017736E-16 ) ) ;
#2234=EDGE_CURVE ( 'NONE', #12385, #752, #7864, .T. ) ;
#2270=ORIENTED_EDGE ( 'NONE', *, *, #3722, .F. ) ;
#2273=DIRECTION ( 'NONE',  ( 6.158143864569485777E-17, 2.736152283717910599E-16, -1.000000000000000000 ) ) ;
#2281=LINE ( 'NONE', #4240, #2080 ) ;
#2283=DIRECTION ( 'NONE',  ( -1.000000000000000000, 0.000000000000000000, 0.000000000000000000 ) ) ;
#2286=ORIENTED_EDGE ( 'NONE', *, *, #5233, .F. ) ;
#2291=DIRECTION ( 'NONE',  ( 0.9960067511297464593, -0.08927794634716622324, 3.401418580343279473E-17 ) ) ;
#2295=DIRECTION ( 'NONE',  ( -6.158143864569485777E-17, -2.736152283717910599E-16, 1.000000000000000000 ) ) ;
#2306=ORIENTED_EDGE ( 'NONE', *, *, #10963, .F. ) ;
#2307=ORIENTED_EDGE ( 'NONE', *, *, #1291, .T. ) ;
#2309=EDGE_CURVE ( 'NONE', #7723, #12373, #2452, .T. ) ;
#2311=AXIS2_PLACEMENT_3D ( 'NONE', #7450, #13745, #13810 ) ;
#2321=DIRECTION ( 'NONE',  ( -1.000000000000000000, 0.000000000000000000, 0.000000000000000000 ) ) ;
#2325=CIRCLE ( 'NONE', #3903, 25.50000000002549783 ) ;
#2329=ORIENTED_EDGE ( 'NONE', *, *, #10705, .T. ) ;
#2339=DIRECTION ( 'NONE',  ( 0.9960067511297464593, -0.08927794634716622324, 3.401418580343279473E-17 ) ) ;
#2346=VECTOR ( 'NONE', #9571, 1000.000000000000000 ) ;
#2347=EDGE_CURVE ( 'NONE', #7744, #11376, #10158, .T. ) ;
#2351=PRODUCT_CONTEXT ( 'NONE', #6296, 'mechanical' ) ;
#2358=CARTESIAN_POINT ( 'NONE',  ( 34.99999999999958789, 1.104930248025249758E-13, -2.499999999999999112 ) ) ;
#2360=ORIENTED_EDGE ( 'NONE', *, *, #2888, .F. ) ;
#2365=ORIENTED_EDGE ( 'NONE', *, *, #5398, .T. ) ;
#2371=LINE ( 'NONE', #4336, #12454 ) ;
#2373=VERTEX_POINT ( 'NONE', #5805 ) ;
#2377=ADVANCED_FACE ( 'NONE', ( #9105 ), #10084, .T. ) ;
#2380=DIRECTION ( 'NONE',  ( 6.158143864569485777E-17, 2.736152283717910599E-16, -1.000000000000000000 ) ) ;
#2382=DIRECTION ( 'NONE',  ( -6.158143864569485777E-17, -2.736152283717910599E-16, 1.000000000000000000 ) ) ;
#2390=DIRECTION ( 'NONE',  ( -6.158143864569485777E-17, -2.736152283717910599E-16, 1.000000000000000000 ) ) ;
#2394=CARTESIAN_POINT ( 'NONE',  ( 34.99999999999958789, 1.091249486606660213E-13, 2.500000000000000000 ) ) ;
#2401=ORIENTED_EDGE ( 'NONE', *, *, #8816, .T. ) ;
#2421=ORIENTED_EDGE ( 'NONE', *, *, #7901, .F. ) ;
#2427=FACE_OUTER_BOUND ( 'NONE', #2968, .T. ) ;
#2445=DIRECTION ( 'NONE',  ( -6.158143864569485777E-17, -2.736152283717910599E-16, 1.000000000000000000 ) ) ;
#2452=CIRCLE ( 'NONE', #10086, 18.74900000001875355 ) ;
#2456=LINE ( 'NONE', #7710, #13496 ) ;
#2457=ORIENTED_EDGE ( 'NONE', *, *, #5172, .F. ) ;
#2458=FACE_OUTER_BOUND ( 'NONE', #9704, .T. ) ;
#2469=AXIS2_PLACEMENT_3D ( 'NONE', #6078, #1728, #1661 ) ;
#2475=CIRCLE ( 'NONE', #12342, 9.000000000009000800 ) ;
#2483=VERTEX_POINT ( 'NONE', #13697 ) ;
#2484=CARTESIAN_POINT ( 'NONE',  ( 52.26118412238654543, 18.64354822589355365, -2.499999999999993339 ) ) ;
#2495=CIRCLE ( 'NONE', #6514, 18.74900000001875000 ) ;
#2502=EDGE_CURVE ( 'NONE', #3802, #3703, #12744, .T. ) ;
#2506=ORIENTED_EDGE ( 'NONE', *, *, #614, .T. ) ;
#2510=PRODUCT_DEFINITION_CONTEXT ( 'detailed design', #6476, 'design' ) ;
#2524=DIRECTION ( 'NONE',  ( 0.9960067511297463483, -0.08927794634716618161, 4.818676322152979407E-17 ) ) ;
#2525=VERTEX_POINT ( 'NONE', #3061 ) ;
#2539=DIRECTION ( 'NONE',  ( 0.9556796851544553384, -0.2944084567112177364, -2.313087999326726136E-17 ) ) ;
#2544=LINE ( 'NONE', #391, #7505 ) ;
#2545=EDGE_LOOP ( 'NONE', ( #13617, #11607, #13883, #11218 ) ) ;
#2552=CARTESIAN_POINT ( 'NONE',  ( 34.99999999999958789, 1.063887963769481123E-13, 12.50000000000000000 ) ) ;
#2553=CYLINDRICAL_SURFACE ( 'NONE', #10635, 9.000000000008999024 ) ;
#2558=CARTESIAN_POINT ( 'NONE',  ( 155.9864723944028810, -111.6214737678657087, -2.500000000000000000 ) ) ;
#2566=DIRECTION ( 'NONE',  ( 0.000000000000000000, 0.000000000000000000, 1.000000000000000000 ) ) ;
#2571=CIRCLE ( 'NONE', #12204, 25.50000000002549783 ) ;
#2593=ORIENTED_EDGE ( 'NONE', *, *, #8742, .F. ) ;
#2594=CARTESIAN_POINT ( 'NONE',  ( 13.76342357120274862, 14.11587126553562221, -2.499999999999996447 ) ) ;
#2603=VECTOR ( 'NONE', #3421, 1000.000000000000000 ) ;
#2606=CIRCLE ( 'NONE', #11072, 9.000000000009000800 ) ;
#2611=AXIS2_PLACEMENT_3D ( 'NONE', #12958, #5503, #6770 ) ;
#2619=DIRECTION ( 'NONE',  ( -6.158143864569485777E-17, -2.736152283717910599E-16, 1.000000000000000000 ) ) ;
#2620=ORIENTED_EDGE ( 'NONE', *, *, #4650, .F. ) ;
#2628=ORIENTED_EDGE ( 'NONE', *, *, #124, .T. ) ;
#2631=VERTEX_POINT ( 'NONE', #186 ) ;
#2633=DIRECTION ( 'NONE',  ( -6.158143864569485777E-17, -2.736152283717910599E-16, 1.000000000000000000 ) ) ;
#2634=DIRECTION ( 'NONE',  ( -6.158143864569485777E-17, -2.736152283717910599E-16, 1.000000000000000000 ) ) ;
#2635=DIRECTION ( 'NONE',  ( 0.1928999275155751925, 0.9812184353977893014, 2.891205793291787151E-16 ) ) ;
#2636=DIRECTION ( 'NONE',  ( -6.158143864569485777E-17, -2.736152283717910599E-16, 1.000000000000000000 ) ) ;
#2643=ORIENTED_EDGE ( 'NONE', *, *, #12535, .T. ) ;
#2645=SHAPE_DEFINITION_REPRESENTATION ( #5400, #12318 ) ;
#2651=CARTESIAN_POINT ( 'NONE',  ( 34.99999999999958789, 1.091249486606660213E-13, 2.500000000000000000 ) ) ;
#2656=VECTOR ( 'NONE', #12777, 1000.000000000000000 ) ;
#2671=CARTESIAN_POINT ( 'NONE',  ( 34.99999999999958789, 1.091249486606660213E-13, 2.500000000000000000 ) ) ;
#2692=DIRECTION ( 'NONE',  ( -0.7328050451781167318, -0.6804386568688601811, -2.409338161076489703E-16 ) ) ;
#2698=CARTESIAN_POINT ( 'NONE',  ( 39.08445607832919677, 20.74481184150345214, -2.499999999999992895 ) ) ;
#2702=DIRECTION ( 'NONE',  ( -6.158143864569485777E-17, -2.736152283717910599E-16, 1.000000000000000000 ) ) ;
#2729=VERTEX_POINT ( 'NONE', #1719 ) ;
#2734=EDGE_LOOP ( 'NONE', ( #1243, #12687, #10659, #9162 ) ) ;
#2739=DIRECTION ( 'NONE',  ( -6.158143864569485777E-17, -2.736152283717910599E-16, 1.000000000000000000 ) ) ;
#2754=CYLINDRICAL_SURFACE ( 'NONE', #10212, 9.000000000008999024 ) ;
#2764=ORIENTED_EDGE ( 'NONE', *, *, #12628, .F. ) ;
#2769=DIRECTION ( 'NONE',  ( -6.158143864569485777E-17, -2.736152283717910599E-16, 1.000000000000000000 ) ) ;
#2771=DIRECTION ( 'NONE',  ( -6.158143864569485777E-17, -2.736152283717910599E-16, 1.000000000000000000 ) ) ;
#2772=ORIENTED_EDGE ( 'NONE', *, *, #5963, .F. ) ;
#2773=LINE ( 'NONE', #544, #2804 ) ;
#2780=AXIS2_PLACEMENT_3D ( 'NONE', #9766, #10741, #7656 ) ;
#2782=ORIENTED_EDGE ( 'NONE', *, *, #1772, .F. ) ;
#2786=ORIENTED_EDGE ( 'NONE', *, *, #7997, .F. ) ;
#2804=VECTOR ( 'NONE', #1848, 1000.000000000000227 ) ;
#2833=CARTESIAN_POINT ( 'NONE',  ( 27.45605056404223987, 17.16431845161426040, -2.499999999999994671 ) ) ;
#2844=EDGE_CURVE ( 'NONE', #1473, #3310, #4071, .T. ) ;
#2848=CIRCLE ( 'NONE', #12484, 18.74900000001875355 ) ;
#2850=ORIENTED_EDGE ( 'NONE', *, *, #7901, .T. ) ;
#2860=VERTEX_POINT ( 'NONE', #11014 ) ;
#2865=ADVANCED_FACE ( 'NONE', ( #7866 ), #12502, .T. ) ;
#2871=CARTESIAN_POINT ( 'NONE',  ( 34.66997162884352690, 21.14050806081579736, -2.499999999999992895 ) ) ;
#2874=CARTESIAN_POINT ( 'NONE',  ( 18.71826692230518674, -9.296782722394514309, -2.500000000000002665 ) ) ;
#2876=EDGE_LOOP ( 'NONE', ( #2772, #12008, #8509, #8883 ) ) ;
#2881=ORIENTED_EDGE ( 'NONE', *, *, #5572, .T. ) ;
#2883=ORIENTED_EDGE ( 'NONE', *, *, #3693, .F. ) ;
#2888=EDGE_CURVE ( 'NONE', #3846, #7956, #11004, .T. ) ;
#2893=DIRECTION ( 'NONE',  ( 0.9960067511297464593, -0.08927794634716622324, 3.401418580343279473E-17 ) ) ;
#2898=DIRECTION ( 'NONE',  ( -0.3926913852462015631, -0.9196703082917374594, -2.775705599192072719E-16 ) ) ;
#2914=DIRECTION ( 'NONE',  ( 0.9928035427100112553, 0.1197544386753605361, 9.637352644305958814E-17 ) ) ;
#2930=ADVANCED_FACE ( 'NONE', ( #1062 ), #7429, .T. ) ;
#2944=DIRECTION ( 'NONE',  ( -0.3926913852462015631, -0.9196703082917374594, -2.775705599192072719E-16 ) ) ;
#2949=VERTEX_POINT ( 'NONE', #6146 ) ;
#2951=AXIS2_PLACEMENT_3D ( 'NONE', #4288, #8568, #3234 ) ;
#2963=DIRECTION ( 'NONE',  ( -6.158143864569485777E-17, -2.736152283717910599E-16, 1.000000000000000000 ) ) ;
#2966=DIRECTION ( 'NONE',  ( 6.158143864569485777E-17, 2.736152283717910599E-16, -1.000000000000000000 ) ) ;
#2968=EDGE_LOOP ( 'NONE', ( #11431, #4933, #5782, #12981 ) ) ;
#2972=DIRECTION ( 'NONE',  ( 0.9960067511297463483, -0.08927794634716620936, 4.626175998653454121E-17 ) ) ;
#3009=ORIENTED_EDGE ( 'NONE', *, *, #352, .F. ) ;
#3011=ORIENTED_EDGE ( 'NONE', *, *, #517, .F. ) ;
#3015=EDGE_CURVE ( 'NONE', #3108, #11568, #11601, .T. ) ;
#3021=AXIS2_PLACEMENT_3D ( 'NONE', #7463, #1165, #51 ) ;
#3029=DIRECTION ( 'NONE',  ( 0.9928035427100113663, 0.1197544386753605777, 9.252351997306908241E-17 ) ) ;
#3031=CARTESIAN_POINT ( 'NONE',  ( 34.99999999999958789, 1.091249486606660213E-13, 2.500000000000000000 ) ) ;
#3046=CARTESIAN_POINT ( 'NONE',  ( 58.70736094381068426, -9.392073098158826738, -2.500000000000000000 ) ) ;
#3055=LINE ( 'NONE', #8651, #1683 ) ;
#3061=CARTESIAN_POINT ( 'NONE',  ( 58.40844909094411719, 10.11407490371516182, 2.500000000000004441 ) ) ;
#3069=DIRECTION ( 'NONE',  ( -6.158143864569485777E-17, -2.736152283717910599E-16, 1.000000000000000000 ) ) ;
#3082=VERTEX_POINT ( 'NONE', #12307 ) ;
#3083=FACE_OUTER_BOUND ( 'NONE', #1608, .T. ) ;
#3086=CARTESIAN_POINT ( 'NONE',  ( 34.99999999999958789, 1.091249486606660213E-13, 2.500000000000000000 ) ) ;
#3088=CARTESIAN_POINT ( 'NONE',  ( 10.11726280447958182, 5.576682675210010487, -2.499999999999999112 ) ) ;
#3090=ADVANCED_FACE ( 'NONE', ( #8027 ), #12907, .T. ) ;
#3093=EDGE_CURVE ( 'NONE', #7898, #11376, #12141, .T. ) ;
#3094=VERTEX_POINT ( 'NONE', #8893 ) ;
#3100=LINE ( 'NONE', #6206, #586 ) ;
#3104=LINE ( 'NONE', #7246, #822 ) ;
#3108=VERTEX_POINT ( 'NONE', #8752 ) ;
#3113=VERTEX_POINT ( 'NONE', #3416 ) ;
#3128=VECTOR ( 'NONE', #3557, 1000.000000000000000 ) ;
#3129=ORIENTED_EDGE ( 'NONE', *, *, #1642, .F. ) ;
#3131=DIRECTION ( 'NONE',  ( -0.9462100554738961389, -0.3235529800822216639, -1.445602896645893329E-16 ) ) ;
#3144=ORIENTED_EDGE ( 'NONE', *, *, #10130, .T. ) ;
#3145=FACE_OUTER_BOUND ( 'NONE', #7216, .T. ) ;
#3156=VERTEX_POINT ( 'NONE', #2164 ) ;
#3158=ORIENTED_EDGE ( 'NONE', *, *, #6531, .F. ) ;
#3163=EDGE_CURVE ( 'NONE', #2525, #9172, #4260, .T. ) ;
#3165=CARTESIAN_POINT ( 'NONE',  ( 34.99999999999958789, 1.104930248025249758E-13, -2.499999999999999112 ) ) ;
#3180=CARTESIAN_POINT ( 'NONE',  ( 47.69307742500824787, -16.90904448151677286, 2.499999999999996003 ) ) ;
#3181=ORIENTED_EDGE ( 'NONE', *, *, #9673, .T. ) ;
#3182=EDGE_CURVE ( 'NONE', #6151, #6555, #10711, .T. ) ;
#3185=EDGE_LOOP ( 'NONE', ( #1740, #3875, #8359, #13169 ) ) ;
#3198=CIRCLE ( 'NONE', #6134, 9.000000000009000800 ) ;
#3208=CIRCLE ( 'NONE', #2311, 18.74900000001875000 ) ;
#3229=VERTEX_POINT ( 'NONE', #508 ) ;
#3234=DIRECTION ( 'NONE',  ( 0.9556796851544554494, -0.2944084567112178474, 0.000000000000000000 ) ) ;
#3238=CARTESIAN_POINT ( 'NONE',  ( 52.27091746333575628, 18.76074118940758595, 2.500000000000006217 ) ) ;
#3245=ORIENTED_EDGE ( 'NONE', *, *, #12549, .T. ) ;
#3249=CIRCLE ( 'NONE', #4366, 9.000000000008999024 ) ;
#3260=AXIS2_PLACEMENT_3D ( 'NONE', #4239, #5970, #10688 ) ;
#3267=ORIENTED_EDGE ( 'NONE', *, *, #13761, .T. ) ;
#3272=DIRECTION ( 'NONE',  ( -6.158143864569485777E-17, -2.736152283717910599E-16, 1.000000000000000000 ) ) ;
#3277=CARTESIAN_POINT ( 'NONE',  ( 34.99999999999958789, 1.091249486606660213E-13, 2.500000000000000000 ) ) ;
#3278=VERTEX_POINT ( 'NONE', #361 ) ;
#3291=VERTEX_POINT ( 'NONE', #5894 ) ;
#3304=CARTESIAN_POINT ( 'NONE',  ( 52.26118412238654543, 18.64354822589355365, -2.499999999999993339 ) ) ;
#3310=VERTEX_POINT ( 'NONE', #2594 ) ;
#3313=ORIENTED_EDGE ( 'NONE', *, *, #7794, .T. ) ;
#3318=EDGE_CURVE ( 'NONE', #5305, #1178, #12582, .T. ) ;
#3327=CARTESIAN_POINT ( 'NONE',  ( 34.99999999999958789, 1.104930248025249758E-13, -2.499999999999999112 ) ) ;
#3329=AXIS2_PLACEMENT_3D ( 'NONE', #804, #5074, #9283 ) ;
#3333=( NAMED_UNIT ( * ) SI_UNIT ( $, .STERADIAN. ) SOLID_ANGLE_UNIT ( ) );
#3335=VERTEX_POINT ( 'NONE', #13637 ) ;
#3341=CARTESIAN_POINT ( 'NONE',  ( 34.99999999999958789, 1.104930248025249758E-13, -2.499999999999999112 ) ) ;
#3347=VERTEX_POINT ( 'NONE', #13707 ) ;
#3348=EDGE_LOOP ( 'NONE', ( #6645, #12608, #279, #11906 ) ) ;
#3363=CARTESIAN_POINT ( 'NONE',  ( 9.857979974958242408, 4.257796268226279324, 8.673617379884035472E-16 ) ) ;
#3365=CARTESIAN_POINT ( 'NONE',  ( 48.99302833075611119, 12.47878836808090064, -2.499999999999994671 ) ) ;
#3369=CARTESIAN_POINT ( 'NONE',  ( 15.01254563088791372, -15.83514028494776760, -5.204170427930421283E-15 ) ) ;
#3370=CARTESIAN_POINT ( 'NONE',  ( 34.99999999999958789, 1.104930248025249758E-13, -2.499999999999999112 ) ) ;
#3375=CARTESIAN_POINT ( 'NONE',  ( 34.99999999999958789, 1.104930248025249758E-13, -2.499999999999999112 ) ) ;
#3376=CARTESIAN_POINT ( 'NONE',  ( 30.92745768374916082, -20.74715399464528787, -2.500000000000005329 ) ) ;
#3379=DIRECTION ( 'NONE',  ( -6.158143864569485777E-17, -2.736152283717910599E-16, 1.000000000000000000 ) ) ;
#3380=DIRECTION ( 'NONE',  ( 6.158143864569485777E-17, 2.736152283717910599E-16, -1.000000000000000000 ) ) ;
#3385=LINE ( 'NONE', #2484, #4352 ) ;
#3386=CARTESIAN_POINT ( 'NONE',  ( 34.99999999999958789, 1.104930248025249758E-13, -2.499999999999999112 ) ) ;
#3393=DIRECTION ( 'NONE',  ( 0.9960067511297463483, -0.08927794634716620936, 4.626175998653454121E-17 ) ) ;
#3394=FACE_OUTER_BOUND ( 'NONE', #445, .T. ) ;
#3409=ORIENTED_EDGE ( 'NONE', *, *, #10824, .F. ) ;
#3416=CARTESIAN_POINT ( 'NONE',  ( 55.16425081158429577, -10.83695794929873912, -2.500000000000000888 ) ) ;
#3417=AXIS2_PLACEMENT_3D ( 'NONE', #3936, #13851, #1965 ) ;
#3419=CIRCLE ( 'NONE', #4543, 2.500000000000000444 ) ;
#3421=DIRECTION ( 'NONE',  ( -6.158143864569485777E-17, -2.736152283717910599E-16, 1.000000000000000000 ) ) ;
#3424=CARTESIAN_POINT ( 'NONE',  ( 52.82363224725100537, -5.817485239812894449, -2.500000000000000000 ) ) ;
#3428=ORIENTED_EDGE ( 'NONE', *, *, #10419, .F. ) ;
#3429=EDGE_CURVE ( 'NONE', #8021, #11572, #6753, .T. ) ;
#3436=DIRECTION ( 'NONE',  ( -6.158143864569485777E-17, -2.736152283717910599E-16, 1.000000000000000000 ) ) ;
#3437=DIRECTION ( 'NONE',  ( -6.158143864569485777E-17, -2.736152283717910599E-16, 1.000000000000000000 ) ) ;
#3442=EDGE_CURVE ( 'NONE', #9172, #11147, #1504, .T. ) ;
#3450=DIRECTION ( 'NONE',  ( -0.3926913852462016186, -0.9196703082917373484, -2.891205793291787644E-16 ) ) ;
#3463=PLANE ( 'NONE',  #10938 ) ;
#3475=DIRECTION ( 'NONE',  ( 0.9960067511297464593, -0.08927794634716622324, 3.401418580343279473E-17 ) ) ;
#3485=CARTESIAN_POINT ( 'NONE',  ( 41.86252833142972918, 24.55922850786694056, -2.499999999999992450 ) ) ;
#3491=DIRECTION ( 'NONE',  ( 0.9928035427100112553, 0.1197544386753605361, 9.637352644305958814E-17 ) ) ;
#3494=DIRECTION ( 'NONE',  ( -6.158143864569485777E-17, -2.736152283717910599E-16, 1.000000000000000000 ) ) ;
#3512=CARTESIAN_POINT ( 'NONE',  ( 30.92745768374916082, -20.74715399464528787, 2.499999999999993783 ) ) ;
#3514=CARTESIAN_POINT ( 'NONE',  ( 34.99999999999958789, 1.104930248025249758E-13, -2.499999999999999112 ) ) ;
#3524=DIRECTION ( 'NONE',  ( -6.158143864569485777E-17, -2.736152283717910599E-16, 1.000000000000000000 ) ) ;
#3529=CIRCLE ( 'NONE', #13449, 18.74900000001875355 ) ;
#3531=DIRECTION ( 'NONE',  ( -0.9960067511297463483, 0.08927794634716619548, 0.000000000000000000 ) ) ;
#3540=DIRECTION ( 'NONE',  ( 0.9960067511297463483, -0.08927794634716620936, 4.626175998653454121E-17 ) ) ;
#3543=CARTESIAN_POINT ( 'NONE',  ( 35.66405164569891184, -18.73723662690267133, -2.500000000000004441 ) ) ;
#3546=ADVANCED_BREP_SHAPE_REPRESENTATION ( '', ( #7695, #8193 ), #5278 ) ;
#3557=DIRECTION ( 'NONE',  ( -6.158143864569485777E-17, -2.736152283717910599E-16, 1.000000000000000000 ) ) ;
#3560=FACE_OUTER_BOUND ( 'NONE', #7152, .T. ) ;
#3566=AXIS2_PLACEMENT_3D ( 'NONE', #1406, #6661, #10927 ) ;
#3573=DIRECTION ( 'NONE',  ( -0.6001121574638169642, 0.7999158696163758409, 1.927470528861191270E-16 ) ) ;
#3575=DIRECTION ( 'NONE',  ( -6.158143864569485777E-17, -2.736152283717910599E-16, 1.000000000000000000 ) ) ;
#3584=ORIENTED_EDGE ( 'NONE', *, *, #725, .T. ) ;
#3590=FACE_OUTER_BOUND ( 'NONE', #7836, .T. ) ;
#3592=CIRCLE ( 'NONE', #1368, 9.000000000009000800 ) ;
#3596=ORIENTED_EDGE ( 'NONE', *, *, #13870, .T. ) ;
#3597=ORIENTED_EDGE ( 'NONE', *, *, #5751, .T. ) ;
#3605=CARTESIAN_POINT ( 'NONE',  ( 55.99165482216006495, 2.525950835318804266, -2.499999999999997335 ) ) ;
#3608=AXIS2_PLACEMENT_3D ( 'NONE', #3512, #3379, #11022 ) ;
#3617=LINE ( 'NONE', #10079, #9280 ) ;
#3619=ORIENTED_EDGE ( 'NONE', *, *, #11052, .F. ) ;
#3620=CARTESIAN_POINT ( 'NONE',  ( 21.34086416022640265, 21.53318388236929692, 5.637851296924623057E-15 ) ) ;
#3646=CIRCLE ( 'NONE', #7676, 9.000000000008999024 ) ;
#3648=EDGE_LOOP ( 'NONE', ( #5995, #2786, #2881, #9372 ) ) ;
#3650=DIRECTION ( 'NONE',  ( -6.158143864569485777E-17, -2.736152283717910599E-16, 1.000000000000000000 ) ) ;
#3653=DIRECTION ( 'NONE',  ( -6.158143864569485777E-17, -2.736152283717910599E-16, 1.000000000000000000 ) ) ;
#3661=VERTEX_POINT ( 'NONE', #9290 ) ;
#3664=CIRCLE ( 'NONE', #5447, 9.000000000008999024 ) ;
#3666=CARTESIAN_POINT ( 'NONE',  ( 10.00024727050385920, -5.026167870790865244, -2.602085213965210642E-15 ) ) ;
#3667=VECTOR ( 'NONE', #6996, 1000.000000000000000 ) ;
#3668=DIRECTION ( 'NONE',  ( -0.8735848310779960046, 0.4866719047884612293, 9.637352644305955116E-17 ) ) ;
#3677=EDGE_CURVE ( 'NONE', #6892, #11850, #8531, .T. ) ;
#3693=EDGE_CURVE ( 'NONE', #4918, #5054, #13525, .T. ) ;
#3703=VERTEX_POINT ( 'NONE', #10605 ) ;
#3704=CARTESIAN_POINT ( 'NONE',  ( 32.05482125692310547, -25.32934902781011743, 2.499999999999992895 ) ) ;
#3708=AXIS2_PLACEMENT_3D ( 'NONE', #5262, #10397, #7097 ) ;
#3720=COLOUR_RGB ( '', 0.31764706, 0.68627451, 0.89019608) ;
#3722=EDGE_CURVE ( 'NONE', #12269, #5851, #6468, .T. ) ;
#3723=ORIENTED_EDGE ( 'NONE', *, *, #8755, .T. ) ;
#3727=CARTESIAN_POINT ( 'NONE',  ( 13.76342357120274862, 14.11587126553561689, 3.035766082959412415E-15 ) ) ;
#3736=DIRECTION ( 'NONE',  ( -6.158143864569485777E-17, -2.736152283717910599E-16, 1.000000000000000000 ) ) ;
#3746=ORIENTED_EDGE ( 'NONE', *, *, #8431, .F. ) ;
#3755=ORIENTED_EDGE ( 'NONE', *, *, #13436, .F. ) ;
#3763=LINE ( 'NONE', #8046, #6821 ) ;
#3770=AXIS2_PLACEMENT_3D ( 'NONE', #11498, #9468, #8406 ) ;
#3780=EDGE_CURVE ( 'NONE', #11568, #1753, #8542, .T. ) ;
#3797=DIRECTION ( 'NONE',  ( -6.158143864569485777E-17, -2.736152283717910599E-16, 1.000000000000000000 ) ) ;
#3800=CYLINDRICAL_SURFACE ( 'NONE', #1246, 25.50000000002549783 ) ;
#3802=VERTEX_POINT ( 'NONE', #6815 ) ;
#3809=EDGE_CURVE ( 'NONE', #5305, #11568, #10766, .T. ) ;
#3812=CARTESIAN_POINT ( 'NONE',  ( 16.29599561779310335, 1.298160649189404880, -2.500000000000000000 ) ) ;
#3819=CIRCLE ( 'NONE', #10528, 9.000000000008999024 ) ;
#3825=DIRECTION ( 'NONE',  ( 0.9960067511297463483, -0.08927794634716618161, 4.818676322152979407E-17 ) ) ;
#3831=ORIENTED_EDGE ( 'NONE', *, *, #723, .F. ) ;
#3832=VERTEX_POINT ( 'NONE', #1272 ) ;
#3842=EDGE_CURVE ( 'NONE', #13800, #4918, #4350, .T. ) ;
#3846=VERTEX_POINT ( 'NONE', #5409 ) ;
#3848=CARTESIAN_POINT ( 'NONE',  ( 15.01254563088791372, -15.83514028494776760, 2.499999999999994227 ) ) ;
#3852=EDGE_CURVE ( 'NONE', #2373, #12385, #4745, .T. ) ;
#3862=ORIENTED_EDGE ( 'NONE', *, *, #12628, .T. ) ;
#3868=CYLINDRICAL_SURFACE ( 'NONE', #1711, 20.00000000000001066 ) ;
#3874=ORIENTED_EDGE ( 'NONE', *, *, #101, .F. ) ;
#3875=ORIENTED_EDGE ( 'NONE', *, *, #4269, .T. ) ;
#3879=EDGE_CURVE ( 'NONE', #4054, #11500, #7791, .T. ) ;
#3884=VECTOR ( 'NONE', #11911, 1000.000000000000000 ) ;
#3886=ORIENTED_EDGE ( 'NONE', *, *, #12722, .T. ) ;
#3892=CARTESIAN_POINT ( 'NONE',  ( 27.98552063842490867, -17.38741154648219833, 2.499999999999994671 ) ) ;
#3899=EDGE_LOOP ( 'NONE', ( #4503, #3009, #1282, #608, #736, #13401, #1878, #3746, #8517, #1900, #4880, #3619, #12912, #8246, #10746, #10220, #2620, #10282, #8813, #2457, #13050, #7992, #12705, #10167, #1057, #4302, #353, #7502, #9330, #6528, #11066, #8691, #800, #9969, #4794, #5319, #8885, #825, #1978, #13860, #6393, #163, #4340, #3158, #4134, #11804, #7858, #5668, #3918, #13142, #5511, #13204, #6989, #8585, #10895, #10509, #10775, #8910, #9724, #13051, #10231, #3755 ) ) ;
#3900=FACE_OUTER_BOUND ( 'NONE', #9554, .T. ) ;
#3903=AXIS2_PLACEMENT_3D ( 'NONE', #11704, #490, #6 ) ;
#3906=CARTESIAN_POINT ( 'NONE',  ( 40.87368016229836343, -22.78235879061917046, -2.500000000000003109 ) ) ;
#3911=CIRCLE ( 'NONE', #12882, 9.000000000009002576 ) ;
#3918=ORIENTED_EDGE ( 'NONE', *, *, #6039, .F. ) ;
#3931=AXIS2_PLACEMENT_3D ( 'NONE', #5331, #10658, #6455 ) ;
#3936=CARTESIAN_POINT ( 'NONE',  ( 26.69171018101576465, -19.44228176112429551, -2.500000000000004441 ) ) ;
#3941=DIRECTION ( 'NONE',  ( 6.158143864569485777E-17, 2.736152283717910599E-16, -1.000000000000000000 ) ) ;
#3947=ORIENTED_EDGE ( 'NONE', *, *, #12796, .T. ) ;
#3957=DIRECTION ( 'NONE',  ( -6.158143864569485777E-17, -2.736152283717910599E-16, 1.000000000000000000 ) ) ;
#3959=ADVANCED_FACE ( 'NONE', ( #8700 ), #13004, .T. ) ;
#3961=ADVANCED_FACE ( 'NONE', ( #9975 ), #4496, .T. ) ;
#3962=FACE_OUTER_BOUND ( 'NONE', #4283, .T. ) ;
#3973=FACE_OUTER_BOUND ( 'NONE', #11628, .T. ) ;
#3989=CIRCLE ( 'NONE', #12284, 9.000000000009002576 ) ;
#3991=EDGE_LOOP ( 'NONE', ( #6431, #216, #13214, #2307 ) ) ;
#4002=CARTESIAN_POINT ( 'NONE',  ( 34.99999999999958789, 1.104930248025249758E-13, -2.499999999999999112 ) ) ;
#4013=DIRECTION ( 'NONE',  ( -0.3926913852462017296, -0.9196703082917372374, -2.891205793291787151E-16 ) ) ;
#4015=ORIENTED_EDGE ( 'NONE', *, *, #5172, .T. ) ;
#4024=EDGE_CURVE ( 'NONE', #11470, #12949, #6028, .T. ) ;
#4025=ADVANCED_FACE ( 'NONE', ( #1552 ), #9268, .T. ) ;
#4027=VERTEX_POINT ( 'NONE', #9203 ) ;
#4028=AXIS2_PLACEMENT_3D ( 'NONE', #4375, #3524, #12022 ) ;
#4030=AXIS2_PLACEMENT_3D ( 'NONE', #6004, #674, #6981 ) ;
#4034=AXIS2_PLACEMENT_3D ( 'NONE', #2552, #12159, #11106 ) ;
#4035=DIRECTION ( 'NONE',  ( 0.000000000000000000, 0.000000000000000000, -1.000000000000000000 ) ) ;
#4041=AXIS2_PLACEMENT_3D ( 'NONE', #1467, #2739, #434 ) ;
#4043=DIRECTION ( 'NONE',  ( -0.8735848310779960046, 0.4866719047884612293, 9.637352644305955116E-17 ) ) ;
#4054=VERTEX_POINT ( 'NONE', #5839 ) ;
#4056=CARTESIAN_POINT ( 'NONE',  ( 19.06870874253413461, 13.90050210118286067, 2.500000000000003109 ) ) ;
#4057=CARTESIAN_POINT ( 'NONE',  ( 52.27091746333575628, 18.76074118940758595, 6.505213034913026604E-15 ) ) ;
#4070=CARTESIAN_POINT ( 'NONE',  ( 53.14943414785363984, 10.84564612680554241, -2.499999999999994671 ) ) ;
#4071=CIRCLE ( 'NONE', #6533, 25.50000000002549783 ) ;
#4078=EDGE_LOOP ( 'NONE', ( #10109, #7156 ) ) ;
#4081=DIRECTION ( 'NONE',  ( -6.158143864569485777E-17, -2.736152283717910599E-16, 1.000000000000000000 ) ) ;
#4082=CIRCLE ( 'NONE', #6548, 25.50000000002549783 ) ;
#4084=CARTESIAN_POINT ( 'NONE',  ( 13.94188849117746010, 1.893657697999893808, -2.500000000000000000 ) ) ;
#4087=DIRECTION ( 'NONE',  ( -6.158143864569485777E-17, -2.736152283717910599E-16, 1.000000000000000000 ) ) ;
#4093=CYLINDRICAL_SURFACE ( 'NONE', #45, 9.000000000008999024 ) ;
#4097=VECTOR ( 'NONE', #1269, 1000.000000000000114 ) ;
#4102=CARTESIAN_POINT ( 'NONE',  ( 34.99999999999958789, 1.063887963769481123E-13, 12.50000000000000000 ) ) ;
#4105=AXIS2_PLACEMENT_3D ( 'NONE', #11575, #13724, #12499 ) ;
#4117=EDGE_CURVE ( 'NONE', #3094, #8676, #8936, .T. ) ;
#4118=DIRECTION ( 'NONE',  ( 0.01532218268401990685, -0.9998826084685129567, -2.775705599192072226E-16 ) ) ;
#4133=CIRCLE ( 'NONE', #9981, 25.50000000002549783 ) ;
#4134=ORIENTED_EDGE ( 'NONE', *, *, #1401, .F. ) ;
#4143=AXIS2_PLACEMENT_3D ( 'NONE', #8858, #9989, #8940 ) ;
#4146=PLANE ( 'NONE',  #4243 ) ;
#4156=CARTESIAN_POINT ( 'NONE',  ( 34.99999999999958789, 1.228057239789091624E-13, -47.50005079999998969 ) ) ;
#4160=ORIENTED_EDGE ( 'NONE', *, *, #7544, .T. ) ;
#4167=CARTESIAN_POINT ( 'NONE',  ( 155.9864723944028810, -111.6214737678657087, -2.500000000000000000 ) ) ;
#4172=CARTESIAN_POINT ( 'NONE',  ( 50.89489709276795537, 9.943703908052050622, 2.500000000000003997 ) ) ;
#4174=CARTESIAN_POINT ( 'NONE',  ( 22.00707094244967621, -21.94159963418280057, -6.505213034913026604E-15 ) ) ;
#4175=EDGE_CURVE ( 'NONE', #13094, #4673, #10040, .T. ) ;
#4176=CIRCLE ( 'NONE', #10450, 9.000000000009002576 ) ;
#4178=( NAMED_UNIT ( * ) SI_UNIT ( $, .STERADIAN. ) SOLID_ANGLE_UNIT ( ) );
#4185=CARTESIAN_POINT ( 'NONE',  ( 60.49844721164429728, -0.2814068163155462599, 1.734723475976807094E-15 ) ) ;
#4188=EDGE_CURVE ( 'NONE', #3291, #11147, #5548, .T. ) ;
#4189=ORIENTED_EDGE ( 'NONE', *, *, #3015, .F. ) ;
#4192=ORIENTED_EDGE ( 'NONE', *, *, #10824, .T. ) ;
#4194=VERTEX_POINT ( 'NONE', #6384 ) ;
#4198=CARTESIAN_POINT ( 'NONE',  ( 75.98647239440286683, -111.6214737678657087, -2.500000000000000000 ) ) ;
#4200=AXIS2_PLACEMENT_3D ( 'NONE', #153, #6651, #11908 ) ;
#4205=VERTEX_POINT ( 'NONE', #4198 ) ;
#4211=AXIS2_PLACEMENT_3D ( 'NONE', #6599, #5691, #6665 ) ;
#4212=EDGE_CURVE ( 'NONE', #2032, #11251, #3529, .T. ) ;
#4213=CARTESIAN_POINT ( 'NONE',  ( 34.99999999999958789, 1.091249486606660213E-13, 2.500000000000000000 ) ) ;
#4223=CIRCLE ( 'NONE', #9834, 18.74900000001875355 ) ;
#4228=EDGE_CURVE ( 'NONE', #7931, #1659, #13877, .T. ) ;
#4232=EDGE_LOOP ( 'NONE', ( #1429, #4677, #7238, #10420 ) ) ;
#4239=CARTESIAN_POINT ( 'NONE',  ( 34.99999999999958789, 1.091249486606660213E-13, 2.500000000000000000 ) ) ;
#4240=CARTESIAN_POINT ( 'NONE',  ( 31.28009342530033265, 25.22721338310705264, 7.806255641895631925E-15 ) ) ;
#4241=AXIS2_PLACEMENT_3D ( 'NONE', #7045, #2633, #13475 ) ;
#4243=AXIS2_PLACEMENT_3D ( 'NONE', #12719, #5508, #2283 ) ;
#4244=CIRCLE ( 'NONE', #687, 9.000000000008999024 ) ;
#4249=CARTESIAN_POINT ( 'NONE',  ( 57.84299132690245671, 11.33347904398042871, 5.204170427930421283E-15 ) ) ;
#4250=CYLINDRICAL_SURFACE ( 'NONE', #12200, 18.74900000001875000 ) ;
#4257=VERTEX_POINT ( 'NONE', #5062 ) ;
#4259=ORIENTED_EDGE ( 'NONE', *, *, #6202, .T. ) ;
#4260=CIRCLE ( 'NONE', #6298, 25.50000000002549783 ) ;
#4263=VERTEX_POINT ( 'NONE', #13787 ) ;
#4269=EDGE_CURVE ( 'NONE', #12738, #7898, #8422, .T. ) ;
#4270=CARTESIAN_POINT ( 'NONE',  ( 34.99999999999958789, 1.104930248025249758E-13, -2.499999999999999112 ) ) ;
#4283=EDGE_LOOP ( 'NONE', ( #3723, #6922, #3584, #899 ) ) ;
#4287=DIRECTION ( 'NONE',  ( 6.158143864569485777E-17, 2.736152283717910599E-16, -1.000000000000000000 ) ) ;
#4288=CARTESIAN_POINT ( 'NONE',  ( 39.71817523509052705, -20.60992048131556942, 2.499999999999994671 ) ) ;
#4294=ADVANCED_FACE ( 'NONE', ( #5673 ), #7764, .T. ) ;
#4295=DIRECTION ( 'NONE',  ( 6.158143864569485777E-17, 2.736152283717910599E-16, -1.000000000000000000 ) ) ;
#4297=AXIS2_PLACEMENT_3D ( 'NONE', #7006, #11562, #10162 ) ;
#4299=CARTESIAN_POINT ( 'NONE',  ( 34.99999999999958789, 1.104930248025249758E-13, -2.499999999999999112 ) ) ;
#4302=ORIENTED_EDGE ( 'NONE', *, *, #2844, .F. ) ;
#4304=VERTEX_POINT ( 'NONE', #8821 ) ;
#4315=DIRECTION ( 'NONE',  ( -6.158143864569485777E-17, -2.736152283717910599E-16, 1.000000000000000000 ) ) ;
#4328=ORIENTED_EDGE ( 'NONE', *, *, #458, .T. ) ;
#4336=CARTESIAN_POINT ( 'NONE',  ( 23.18128365339294916, -22.59575057217061556, -6.505213034913026604E-15 ) ) ;
#4338=CIRCLE ( 'NONE', #6162, 9.000000000009000800 ) ;
#4340=ORIENTED_EDGE ( 'NONE', *, *, #8325, .F. ) ;
#4342=ADVANCED_FACE ( 'NONE', ( #6449 ), #7632, .T. ) ;
#4346=DIRECTION ( 'NONE',  ( 0.9960067511297464593, -0.08927794634716622324, 6.802837160686558945E-17 ) ) ;
#4348=CARTESIAN_POINT ( 'NONE',  ( 43.29712336220986657, 19.44704974301885159, -2.499999999999993783 ) ) ;
#4350=LINE ( 'NONE', #1153, #12365 ) ;
#4352=VECTOR ( 'NONE', #6760, 1000.000000000000000 ) ;
#4361=DIRECTION ( 'NONE',  ( 0.000000000000000000, 0.000000000000000000, -1.000000000000000000 ) ) ;
#4366=AXIS2_PLACEMENT_3D ( 'NONE', #9492, #11658, #8497 ) ;
#4375=CARTESIAN_POINT ( 'NONE',  ( 19.50211115783503857, -14.38212227840833179, -2.500000000000004441 ) ) ;
#4386=SHAPE_REPRESENTATION_RELATIONSHIP ( 'NONE' , 'NONE' ,  #12318, #3546 ) ;
#4391=VECTOR ( 'NONE', #13493, 1000.000000000000000 ) ;
#4400=DIRECTION ( 'NONE',  ( 0.9960067511297464593, -0.08927794634716622324, 3.401418580343279473E-17 ) ) ;
#4409=ORIENTED_EDGE ( 'NONE', *, *, #6195, .F. ) ;
#4416=DIRECTION ( 'NONE',  ( 0.4206864060305147146, -0.9072061219927525233, -2.409338161076489703E-16 ) ) ;
#4432=VERTEX_POINT ( 'NONE', #13063 ) ;
#4436=CARTESIAN_POINT ( 'NONE',  ( 34.99999999999958789, 1.104930248025249758E-13, -2.499999999999999112 ) ) ;
#4437=EDGE_CURVE ( 'NONE', #3113, #6530, #7696, .T. ) ;
#4442=CARTESIAN_POINT ( 'NONE',  ( 60.49844721164429728, -0.2814068163155470925, 2.500000000000001332 ) ) ;
#4449=( NAMED_UNIT ( * ) PLANE_ANGLE_UNIT ( ) SI_UNIT ( $, .RADIAN. ) );
#4456=CIRCLE ( 'NONE', #7378, 9.000000000009002576 ) ;
#4463=VECTOR ( 'NONE', #12503, 1000.000000000000114 ) ;
#4473=EDGE_CURVE ( 'NONE', #4673, #7723, #8977, .T. ) ;
#4483=CIRCLE ( 'NONE', #12105, 9.000000000008999024 ) ;
#4484=EDGE_LOOP ( 'NONE', ( #13038, #1541, #520, #3862 ) ) ;
#4493=AXIS2_PLACEMENT_3D ( 'NONE', #4619, #13770, #11620 ) ;
#4496=CYLINDRICAL_SURFACE ( 'NONE', #4211, 9.000000000008999024 ) ;
#4500=DIRECTION ( 'NONE',  ( 0.9960067511297463483, -0.08927794634716619548, 0.000000000000000000 ) ) ;
#4503=ORIENTED_EDGE ( 'NONE', *, *, #2502, .F. ) ;
#4504=DIRECTION ( 'NONE',  ( -6.158143864569485777E-17, -2.736152283717910599E-16, 1.000000000000000000 ) ) ;
#4515=FACE_OUTER_BOUND ( 'NONE', #7454, .T. ) ;
#4518=VERTEX_POINT ( 'NONE', #3848 ) ;
#4520=DIRECTION ( 'NONE',  ( -6.158143864569485777E-17, -2.736152283717910599E-16, 1.000000000000000000 ) ) ;
#4524=CIRCLE ( 'NONE', #7013, 18.74900000001875000 ) ;
#4534=CIRCLE ( 'NONE', #7457, 9.000000000008999024 ) ;
#4536=ORIENTED_EDGE ( 'NONE', *, *, #9518, .F. ) ;
#4543=AXIS2_PLACEMENT_3D ( 'NONE', #6408, #4295, #4500 ) ;
#4544=SURFACE_SIDE_STYLE ('',( #5386 ) ) ;
#4554=CARTESIAN_POINT ( 'NONE',  ( 34.99999999999958789, 1.091249486606660213E-13, 2.500000000000000000 ) ) ;
#4570=ORIENTED_EDGE ( 'NONE', *, *, #4437, .T. ) ;
#4571=DIRECTION ( 'NONE',  ( 0.1928999275155749149, 0.9812184353977894125, 2.775705599192072226E-16 ) ) ;
#4579=ORIENTED_EDGE ( 'NONE', *, *, #1463, .F. ) ;
#4593=ORIENTED_EDGE ( 'NONE', *, *, #6132, .T. ) ;
#4597=AXIS2_PLACEMENT_3D ( 'NONE', #9485, #2966, #6055 ) ;
#4603=DIRECTION ( 'NONE',  ( -6.158143864569485777E-17, -2.736152283717910599E-16, 1.000000000000000000 ) ) ;
#4615=ORIENTED_EDGE ( 'NONE', *, *, #6005, .T. ) ;
#4619=CARTESIAN_POINT ( 'NONE',  ( 19.50211115783503857, -14.38212227840833179, 2.499999999999995115 ) ) ;
#4628=ORIENTED_EDGE ( 'NONE', *, *, #7977, .T. ) ;
#4629=EDGE_CURVE ( 'NONE', #576, #8296, #7416, .T. ) ;
#4637=CARTESIAN_POINT ( 'NONE',  ( 34.99999999999958789, 1.091249486606660213E-13, 2.500000000000000000 ) ) ;
#4641=CARTESIAN_POINT ( 'NONE',  ( 34.99999999999958789, 1.063887963769481123E-13, 12.50000000000000000 ) ) ;
#4648=ORIENTED_EDGE ( 'NONE', *, *, #8248, .T. ) ;
#4650=EDGE_CURVE ( 'NONE', #5851, #13160, #12505, .T. ) ;
#4653=CARTESIAN_POINT ( 'NONE',  ( 50.48962708925064646, 14.39101985375337556, 2.500000000000004885 ) ) ;
#4654=CARTESIAN_POINT ( 'NONE',  ( 23.18128365339294916, -22.59575057217061556, 2.499999999999992895 ) ) ;
#4657=DIRECTION ( 'NONE',  ( 0.000000000000000000, 0.000000000000000000, 1.000000000000000000 ) ) ;
#4669=ADVANCED_FACE ( 'NONE', ( #2427 ), #12970, .T. ) ;
#4673=VERTEX_POINT ( 'NONE', #10698 ) ;
#4674=AXIS2_PLACEMENT_3D ( 'NONE', #7023, #3797, #1697 ) ;
#4677=ORIENTED_EDGE ( 'NONE', *, *, #2234, .F. ) ;
#4685=ORIENTED_EDGE ( 'NONE', *, *, #8930, .T. ) ;
#4698=CIRCLE ( 'NONE', #4929, 9.000000000008999024 ) ;
#4709=CIRCLE ( 'NONE', #11429, 9.000000000009002576 ) ;
#4716=AXIS2_PLACEMENT_3D ( 'NONE', #2093, #9794, #13036 ) ;
#4718=ORIENTED_EDGE ( 'NONE', *, *, #686, .T. ) ;
#4719=ORIENTED_EDGE ( 'NONE', *, *, #5840, .F. ) ;
#4720=VERTEX_POINT ( 'NONE', #6568 ) ;
#4738=DIRECTION ( 'NONE',  ( -6.158143864569485777E-17, -2.736152283717910599E-16, 1.000000000000000000 ) ) ;
#4740=DIRECTION ( 'NONE',  ( 0.000000000000000000, 0.000000000000000000, 1.000000000000000000 ) ) ;
#4745=CIRCLE ( 'NONE', #13040, 18.74900000001875000 ) ;
#4750=ORIENTED_EDGE ( 'NONE', *, *, #9597, .F. ) ;
#4757=EDGE_LOOP ( 'NONE', ( #1119, #3428, #4878, #4328 ) ) ;
#4768=CARTESIAN_POINT ( 'NONE',  ( 34.99999999999958789, 1.104930248025249758E-13, -2.499999999999999112 ) ) ;
#4778=ORIENTED_EDGE ( 'NONE', *, *, #614, .F. ) ;
#4794=ORIENTED_EDGE ( 'NONE', *, *, #6178, .F. ) ;
#4799=ORIENTED_EDGE ( 'NONE', *, *, #3722, .T. ) ;
#4803=CARTESIAN_POINT ( 'NONE',  ( 51.25836974494252019, 19.64472991003004054, 2.500000000000006661 ) ) ;
#4814=CYLINDRICAL_SURFACE ( 'NONE', #5073, 9.000000000008999024 ) ;
#4816=EDGE_CURVE ( 'NONE', #3291, #2525, #5806, .T. ) ;
#4832=DIRECTION ( 'NONE',  ( -6.158143864569485777E-17, -2.736152283717910599E-16, 1.000000000000000000 ) ) ;
#4840=ORIENTED_EDGE ( 'NONE', *, *, #744, .T. ) ;
#4843=CARTESIAN_POINT ( 'NONE',  ( 53.02537423504344360, -5.158573900538657497, -2.499999999999999112 ) ) ;
#4845=LINE ( 'NONE', #9120, #2603 ) ;
#4852=DIRECTION ( 'NONE',  ( -6.158143864569485777E-17, -2.736152283717910599E-16, 1.000000000000000000 ) ) ;
#4860=CARTESIAN_POINT ( 'NONE',  ( 42.70768697973989703, 17.09141780026012114, -2.499999999999993783 ) ) ;
#4863=AXIS2_PLACEMENT_3D ( 'NONE', #8456, #8389, #12617 ) ;
#4867=FACE_OUTER_BOUND ( 'NONE', #209, .T. ) ;
#4875=CARTESIAN_POINT ( 'NONE',  ( 14.99223790936468603, -6.835163196276449860, -2.500000000000002665 ) ) ;
#4877=FACE_OUTER_BOUND ( 'NONE', #2734, .T. ) ;
#4878=ORIENTED_EDGE ( 'NONE', *, *, #12549, .F. ) ;
#4880=ORIENTED_EDGE ( 'NONE', *, *, #12452, .F. ) ;
#4886=ADVANCED_FACE ( 'NONE', ( #7330 ), #10291, .T. ) ;
#4890=EDGE_CURVE ( 'NONE', #7032, #534, #4176, .T. ) ;
#4905=ADVANCED_FACE ( 'NONE', ( #4964 ), #13825, .T. ) ;
#4911=VERTEX_POINT ( 'NONE', #6090 ) ;
#4913=EDGE_LOOP ( 'NONE', ( #4750, #2, #6715, #13035 ) ) ;
#4915=AXIS2_PLACEMENT_3D ( 'NONE', #12449, #3957, #9359 ) ;
#4918=VERTEX_POINT ( 'NONE', #4172 ) ;
#4919=LINE ( 'NONE', #3727, #10375 ) ;
#4927=LINE ( 'NONE', #4860, #1250 ) ;
#4929=AXIS2_PLACEMENT_3D ( 'NONE', #1561, #1770, #2692 ) ;
#4933=ORIENTED_EDGE ( 'NONE', *, *, #778, .F. ) ;
#4946=DIRECTION ( 'NONE',  ( 0.9960067511297464593, -0.08927794634716622324, 3.401418580343279473E-17 ) ) ;
#4951=CIRCLE ( 'NONE', #4716, 9.000000000008999024 ) ;
#4959=AXIS2_PLACEMENT_3D ( 'NONE', #10801, #2390, #10939 ) ;
#4964=FACE_OUTER_BOUND ( 'NONE', #3348, .T. ) ;
#4973=CARTESIAN_POINT ( 'NONE',  ( 56.05919550416194141, -1.881564379087038885, 2.500000000000000888 ) ) ;
#4991=CARTESIAN_POINT ( 'NONE',  ( 34.99999999999958789, 1.104930248025249758E-13, -2.499999999999999112 ) ) ;
#4993=DIRECTION ( 'NONE',  ( 0.9960067511297463483, -0.08927794634716620936, 4.626175998653454121E-17 ) ) ;
#4997=DIRECTION ( 'NONE',  ( 0.9960067511297464593, -0.08927794634716622324, 6.802837160686558945E-17 ) ) ;
#5012=DIRECTION ( 'NONE',  ( -6.158143864569485777E-17, -2.736152283717910599E-16, 1.000000000000000000 ) ) ;
#5027=LINE ( 'NONE', #3906, #3667 ) ;
#5030=CARTESIAN_POINT ( 'NONE',  ( 10.29982004912478821, -6.336490384724132952, -2.500000000000002665 ) ) ;
#5037=EDGE_LOOP ( 'NONE', ( #11213, #10722, #9721, #3181 ) ) ;
#5050=AXIS2_PLACEMENT_3D ( 'NONE', #5765, #13454, #13304 ) ;
#5054=VERTEX_POINT ( 'NONE', #8720 ) ;
#5055=CARTESIAN_POINT ( 'NONE',  ( 52.85884796071297131, 5.708463060827149604, -2.499999999999996447 ) ) ;
#5062=CARTESIAN_POINT ( 'NONE',  ( 60.47785218637952198, 1.062566689801824893, 2.500000000000001776 ) ) ;
#5064=DIRECTION ( 'NONE',  ( -0.9960067511297463483, 0.08927794634716620936, -4.818676322152979407E-17 ) ) ;
#5073=AXIS2_PLACEMENT_3D ( 'NONE', #3605, #2636, #412 ) ;
#5074=DIRECTION ( 'NONE',  ( -6.158143864569485777E-17, -2.736152283717910599E-16, 1.000000000000000000 ) ) ;
#5078=DIRECTION ( 'NONE',  ( -6.158143864569485777E-17, -2.736152283717910599E-16, 1.000000000000000000 ) ) ;
#5088=FACE_OUTER_BOUND ( 'NONE', #7462, .T. ) ;
#5090=CARTESIAN_POINT ( 'NONE',  ( 82.09155748149851206, -71.43674177705591433, 2.500000000000000000 ) ) ;
#5098=CARTESIAN_POINT ( 'NONE',  ( 34.99999999999958789, 1.063887963769481123E-13, 12.50000000000000000 ) ) ;
#5102=EDGE_LOOP ( 'NONE', ( #6963, #3129, #756, #2643 ) ) ;
#5114=AXIS2_PLACEMENT_3D ( 'NONE', #335, #7742, #13261 ) ;
#5116=EDGE_LOOP ( 'NONE', ( #7504, #12044, #5593, #6502 ) ) ;
#5118=ORIENTED_EDGE ( 'NONE', *, *, #13773, .F. ) ;
#5122=DIRECTION ( 'NONE',  ( -6.158143864569485777E-17, -2.736152283717910599E-16, 1.000000000000000000 ) ) ;
#5128=ORIENTED_EDGE ( 'NONE', *, *, #9776, .T. ) ;
#5131=FACE_OUTER_BOUND ( 'NONE', #10860, .T. ) ;
#5139=CIRCLE ( 'NONE', #4241, 9.000000000008999024 ) ;
#5144=CARTESIAN_POINT ( 'NONE',  ( 32.05482125692310547, -25.32934902781012099, -2.500000000000006217 ) ) ;
#5147=EDGE_CURVE ( 'NONE', #6243, #3832, #11353, .T. ) ;
#5163=VECTOR ( 'NONE', #1049, 1000.000000000000000 ) ;
#5167=AXIS2_PLACEMENT_3D ( 'NONE', #7107, #740, #12384 ) ;
#5172=EDGE_CURVE ( 'NONE', #1257, #3094, #2848, .T. ) ;
#5176=CARTESIAN_POINT ( 'NONE',  ( 34.99999999999958789, 1.104930248025249758E-13, -2.499999999999999112 ) ) ;
#5188=CARTESIAN_POINT ( 'NONE',  ( 31.28009342530033265, 25.22721338310704908, -2.499999999999992450 ) ) ;
#5192=DIRECTION ( 'NONE',  ( 0.9960067511297464593, -0.08927794634716622324, 6.802837160686558945E-17 ) ) ;
#5202=VERTEX_POINT ( 'NONE', #1656 ) ;
#5203=CARTESIAN_POINT ( 'NONE',  ( 34.99999999999958789, 1.104930248025249758E-13, -2.499999999999999112 ) ) ;
#5206=CARTESIAN_POINT ( 'NONE',  ( 26.69171018101576465, -19.44228176112429551, 2.499999999999994227 ) ) ;
#5208=AXIS2_PLACEMENT_3D ( 'NONE', #11887, #13031, #1174 ) ;
#5209=FACE_OUTER_BOUND ( 'NONE', #9247, .T. ) ;
#5214=DIRECTION ( 'NONE',  ( -6.158143864569485777E-17, -2.736152283717910599E-16, 1.000000000000000000 ) ) ;
#5215=DIRECTION ( 'NONE',  ( -6.158143864569485777E-17, -2.736152283717910599E-16, 1.000000000000000000 ) ) ;
#5217=VERTEX_POINT ( 'NONE', #11580 ) ;
#5233=EDGE_CURVE ( 'NONE', #534, #2631, #1513, .T. ) ;
#5234=ORIENTED_EDGE ( 'NONE', *, *, #12455, .F. ) ;
#5240=ADVANCED_FACE ( 'NONE', ( #12390 ), #1720, .T. ) ;
#5257=DIRECTION ( 'NONE',  ( -0.9960067511297463483, 0.08927794634716618161, -4.818676322152979407E-17 ) ) ;
#5262=CARTESIAN_POINT ( 'NONE',  ( 34.66997162884352690, 21.14050806081579736, -2.499999999999992895 ) ) ;
#5263=CIRCLE ( 'NONE', #7716, 9.000000000008999024 ) ;
#5270=CARTESIAN_POINT ( 'NONE',  ( 22.31663499682298735, 16.91633092580596198, -2.499999999999995559 ) ) ;
#5277=DIRECTION ( 'NONE',  ( 6.158143864569485777E-17, 2.736152283717910599E-16, -1.000000000000000000 ) ) ;
#5278=( GEOMETRIC_REPRESENTATION_CONTEXT ( 3 ) GLOBAL_UNCERTAINTY_ASSIGNED_CONTEXT ( ( #7685 ) ) GLOBAL_UNIT_ASSIGNED_CONTEXT ( ( #8533, #4449, #3333 ) ) REPRESENTATION_CONTEXT ( 'NONE', 'WORKASPACE' ) );
#5290=CARTESIAN_POINT ( 'NONE',  ( 38.24615002434714484, 18.46584715143433542, -2.499999999999993783 ) ) ;
#5301=CARTESIAN_POINT ( 'NONE',  ( 45.47624229149391084, 15.54906262289183871, 2.500000000000004885 ) ) ;
#5303=EDGE_CURVE ( 'NONE', #12212, #3703, #5389, .T. ) ;
#5305=VERTEX_POINT ( 'NONE', #3892 ) ;
#5319=ORIENTED_EDGE ( 'NONE', *, *, #17, .F. ) ;
#5331=CARTESIAN_POINT ( 'NONE',  ( 34.99999999999958789, 1.063887963769481123E-13, 12.50000000000000000 ) ) ;
#5335=EDGE_CURVE ( 'NONE', #3347, #3846, #8617, .T. ) ;
#5350=EDGE_LOOP ( 'NONE', ( #11505, #1771, #11142, #7646 ) ) ;
#5353=ORIENTED_EDGE ( 'NONE', *, *, #9597, .T. ) ;
#5361=FACE_OUTER_BOUND ( 'NONE', #1353, .T. ) ;
#5375=EDGE_CURVE ( 'NONE', #8314, #1753, #11077, .T. ) ;
#5377=ORIENTED_EDGE ( 'NONE', *, *, #9258, .F. ) ;
#5386=SURFACE_STYLE_FILL_AREA ( #5457 ) ;
#5389=LINE ( 'NONE', #6007, #11041 ) ;
#5395=EDGE_CURVE ( 'NONE', #4673, #12017, #5665, .T. ) ;
#5396=ORIENTED_EDGE ( 'NONE', *, *, #5375, .F. ) ;
#5397=VERTEX_POINT ( 'NONE', #3485 ) ;
#5398=EDGE_CURVE ( 'NONE', #5054, #11019, #3198, .T. ) ;
#5400=PRODUCT_DEFINITION_SHAPE ( 'NONE', 'NONE',  #11145 ) ;
#5402=DIRECTION ( 'NONE',  ( -6.158143864569485777E-17, -2.736152283717910599E-16, 1.000000000000000000 ) ) ;
#5404=DIRECTION ( 'NONE',  ( -0.9960067511297463483, 0.08927794634716618161, -4.818676322152979407E-17 ) ) ;
#5409=CARTESIAN_POINT ( 'NONE',  ( 53.56517978609545594, 2.618988451796027572, 2.500000000000001776 ) ) ;
#5413=DIRECTION ( 'NONE',  ( 0.7533101279583153120, -0.6576654553155628635, -1.445602896645893822E-16 ) ) ;
#5416=CARTESIAN_POINT ( 'NONE',  ( 16.53267785980283477, 10.29504797295195750, -2.499999999999997335 ) ) ;
#5438=AXIS2_PLACEMENT_3D ( 'NONE', #7498, #11780, #4946 ) ;
#5447=AXIS2_PLACEMENT_3D ( 'NONE', #5544, #3736, #7027 ) ;
#5450=EDGE_CURVE ( 'NONE', #1473, #11569, #7767, .T. ) ;
#5453=ORIENTED_EDGE ( 'NONE', *, *, #13773, .T. ) ;
#5457=FILL_AREA_STYLE ('',( #288 ) ) ;
#5471=VERTEX_POINT ( 'NONE', #7339 ) ;
#5483=CARTESIAN_POINT ( 'NONE',  ( 42.70768697973989703, 17.09141780026012114, -2.499999999999993783 ) ) ;
#5485=ORIENTED_EDGE ( 'NONE', *, *, #5375, .T. ) ;
#5486=AXIS2_PLACEMENT_3D ( 'NONE', #12160, #2769, #3668 ) ;
#5488=DIRECTION ( 'NONE',  ( -6.158143864569485777E-17, -2.736152283717910599E-16, 1.000000000000000000 ) ) ;
#5497=FACE_OUTER_BOUND ( 'NONE', #13862, .T. ) ;
#5503=DIRECTION ( 'NONE',  ( -6.158143864569485777E-17, -2.736152283717910599E-16, 1.000000000000000000 ) ) ;
#5504=AXIS2_PLACEMENT_3D ( 'NONE', #11515, #858, #3029 ) ;
#5507=STYLED_ITEM ( 'NONE', ( #6363 ), #3546 ) ;
#5508=DIRECTION ( 'NONE',  ( 0.000000000000000000, 0.000000000000000000, -1.000000000000000000 ) ) ;
#5511=ORIENTED_EDGE ( 'NONE', *, *, #6851, .F. ) ;
#5512=DIRECTION ( 'NONE',  ( -6.158143864569485777E-17, -2.736152283717910599E-16, 1.000000000000000000 ) ) ;
#5513=EDGE_CURVE ( 'NONE', #12017, #12373, #6108, .T. ) ;
#5532=ORIENTED_EDGE ( 'NONE', *, *, #7281, .T. ) ;
#5544=CARTESIAN_POINT ( 'NONE',  ( 55.00383357371546822, 6.846651893462920135, -2.499999999999995559 ) ) ;
#5548=CIRCLE ( 'NONE', #1752, 25.50000000002549783 ) ;
#5551=DIRECTION ( 'NONE',  ( -0.2228746399763467390, 0.9748471135800802490, 2.409338161076489210E-16 ) ) ;
#5555=ORIENTED_EDGE ( 'NONE', *, *, #6202, .F. ) ;
#5564=DIRECTION ( 'NONE',  ( 0.9928035427100113663, 0.1197544386753605777, 9.252351997306908241E-17 ) ) ;
#5571=ORIENTED_EDGE ( 'NONE', *, *, #1219, .F. ) ;
#5572=EDGE_CURVE ( 'NONE', #2860, #4027, #4524, .T. ) ;
#5574=CIRCLE ( 'NONE', #4915, 9.000000000008999024 ) ;
#5583=DIRECTION ( 'NONE',  ( -0.7328050451781167318, -0.6804386568688601811, -2.313087999326727184E-16 ) ) ;
#5584=VECTOR ( 'NONE', #4361, 1000.000000000000000 ) ;
#5593=ORIENTED_EDGE ( 'NONE', *, *, #5398, .F. ) ;
#5594=VERTEX_POINT ( 'NONE', #3543 ) ;
#5597=DIRECTION ( 'NONE',  ( -6.158143864569485777E-17, -2.736152283717910599E-16, 1.000000000000000000 ) ) ;
#5644=CARTESIAN_POINT ( 'NONE',  ( 34.99999999999958789, 1.063887963769481123E-13, 12.50000000000000000 ) ) ;
#5645=CARTESIAN_POINT ( 'NONE',  ( 14.00979921278056040, -2.538005261501628862, 2.499999999999997780 ) ) ;
#5665=CIRCLE ( 'NONE', #7918, 18.74900000001875355 ) ;
#5668=ORIENTED_EDGE ( 'NONE', *, *, #4188, .F. ) ;
#5670=EDGE_LOOP ( 'NONE', ( #7711, #9793, #2081, #468 ) ) ;
#5673=FACE_OUTER_BOUND ( 'NONE', #6247, .T. ) ;
#5674=EDGE_CURVE ( 'NONE', #4194, #6463, #7907, .T. ) ;
#5685=CARTESIAN_POINT ( 'NONE',  ( 21.51985683731163945, -13.03114504999992995, -2.500000000000004441 ) ) ;
#5687=DIRECTION ( 'NONE',  ( -6.158143864569485777E-17, -2.736152283717910599E-16, 1.000000000000000000 ) ) ;
#5691=DIRECTION ( 'NONE',  ( -6.158143864569485777E-17, -2.736152283717910599E-16, 1.000000000000000000 ) ) ;
#5704=VERTEX_POINT ( 'NONE', #10293 ) ;
#5730=CIRCLE ( 'NONE', #7984, 25.50000000002549783 ) ;
#5735=EDGE_LOOP ( 'NONE', ( #8767, #10666 ) ) ;
#5739=ORIENTED_EDGE ( 'NONE', *, *, #11843, .T. ) ;
#5751=EDGE_CURVE ( 'NONE', #5471, #6547, #12624, .T. ) ;
#5765=CARTESIAN_POINT ( 'NONE',  ( 34.99999999999958789, 1.091249486606660213E-13, 2.500000000000000000 ) ) ;
#5767=DIRECTION ( 'NONE',  ( 0.9960067511297463483, -0.08927794634716618161, 4.818676322152979407E-17 ) ) ;
#5770=ORIENTED_EDGE ( 'NONE', *, *, #7290, .T. ) ;
#5782=ORIENTED_EDGE ( 'NONE', *, *, #11052, .T. ) ;
#5805=CARTESIAN_POINT ( 'NONE',  ( 21.51985683731163945, -13.03114504999992995, 2.499999999999995559 ) ) ;
#5806=LINE ( 'NONE', #13195, #4391 ) ;
#5808=AXIS2_PLACEMENT_3D ( 'NONE', #10732, #170, #34 ) ;
#5813=VECTOR ( 'NONE', #3436, 1000.000000000000000 ) ;
#5821=DIRECTION ( 'NONE',  ( 0.9960067511297463483, -0.08927794634716619548, 0.000000000000000000 ) ) ;
#5828=AXIS2_PLACEMENT_3D ( 'NONE', #8579, #10479, #881 ) ;
#5832=CARTESIAN_POINT ( 'NONE',  ( 14.99223790936468603, -6.835163196276451636, 2.499999999999996891 ) ) ;
#5836=DIRECTION ( 'NONE',  ( -0.6001121574638170753, 0.7999158696163758409, 1.850470399461381402E-16 ) ) ;
#5839=CARTESIAN_POINT ( 'NONE',  ( 18.71826692230518674, -9.296782722394517862, 2.499999999999996447 ) ) ;
#5840=EDGE_CURVE ( 'NONE', #7540, #4205, #1802, .T. ) ;
#5846=DIRECTION ( 'NONE',  ( -0.9462100554738961389, -0.3235529800822216639, -1.445602896645893329E-16 ) ) ;
#5850=ORIENTED_EDGE ( 'NONE', *, *, #12901, .F. ) ;
#5851=VERTEX_POINT ( 'NONE', #5030 ) ;
#5854=EDGE_LOOP ( 'NONE', ( #4536, #6445, #6552, #5891 ) ) ;
#5859=DIRECTION ( 'NONE',  ( 6.158143864569485777E-17, 2.736152283717910599E-16, -1.000000000000000000 ) ) ;
#5891=ORIENTED_EDGE ( 'NONE', *, *, #8380, .T. ) ;
#5894=CARTESIAN_POINT ( 'NONE',  ( 58.40844909094411719, 10.11407490371516360, -2.499999999999994671 ) ) ;
#5898=CARTESIAN_POINT ( 'NONE',  ( 38.81043356982896597, -18.35771219435081392, 2.499999999999995115 ) ) ;
#5906=ORIENTED_EDGE ( 'NONE', *, *, #352, .T. ) ;
#5907=DIRECTION ( 'NONE',  ( 6.158143864569485777E-17, 2.736152283717910599E-16, -1.000000000000000000 ) ) ;
#5916=EDGE_LOOP ( 'NONE', ( #12639, #5770, #10966, #4192 ) ) ;
#5925=CARTESIAN_POINT ( 'NONE',  ( 45.47624229149391084, 15.54906262289183871, -2.499999999999994671 ) ) ;
#5927=DIRECTION ( 'NONE',  ( -6.158143864569485777E-17, -2.736152283717910599E-16, 1.000000000000000000 ) ) ;
#5935=VECTOR ( 'NONE', #9337, 1000.000000000000000 ) ;
#5938=CARTESIAN_POINT ( 'NONE',  ( 62.16766351966359849, -73.17985663200910551, -2.500000000000000000 ) ) ;
#5963=EDGE_CURVE ( 'NONE', #420, #6463, #2281, .T. ) ;
#5964=ORIENTED_EDGE ( 'NONE', *, *, #4437, .F. ) ;
#5967=AXIS2_PLACEMENT_3D ( 'NONE', #8428, #11517, #4997 ) ;
#5970=DIRECTION ( 'NONE',  ( -6.158143864569485777E-17, -2.736152283717910599E-16, 1.000000000000000000 ) ) ;
#5974=ORIENTED_EDGE ( 'NONE', *, *, #6362, .T. ) ;
#5976=ORIENTED_EDGE ( 'NONE', *, *, #3693, .T. ) ;
#5977=CARTESIAN_POINT ( 'NONE',  ( 30.92745768374916082, -20.74715399464528787, -2.500000000000005329 ) ) ;
#5986=DIRECTION ( 'NONE',  ( -6.158143864569485777E-17, -2.736152283717910599E-16, 1.000000000000000000 ) ) ;
#5995=ORIENTED_EDGE ( 'NONE', *, *, #1816, .F. ) ;
#5999=CARTESIAN_POINT ( 'NONE',  ( 39.08445607832919677, 20.74481184150345214, -2.499999999999992895 ) ) ;
#6003=CARTESIAN_POINT ( 'NONE',  ( 22.84091969677297485, -17.29701610032388359, -2.500000000000004441 ) ) ;
#6004=CARTESIAN_POINT ( 'NONE',  ( 34.99999999999958789, 1.091249486606660213E-13, 2.500000000000000000 ) ) ;
#6005=EDGE_CURVE ( 'NONE', #5594, #2949, #11490, .T. ) ;
#6007=CARTESIAN_POINT ( 'NONE',  ( 76.84607712649204814, -99.92541302764922762, 2.500000000000000000 ) ) ;
#6015=CARTESIAN_POINT ( 'NONE',  ( 17.38503225228318883, -6.421675190136373779, -2.500000000000002665 ) ) ;
#6021=ADVANCED_FACE ( 'NONE', ( #5361 ), #9854, .T. ) ;
#6028=CIRCLE ( 'NONE', #7139, 25.50000000002549783 ) ;
#6030=VERTEX_POINT ( 'NONE', #4442 ) ;
#6039=EDGE_CURVE ( 'NONE', #5217, #3291, #8129, .T. ) ;
#6041=DIRECTION ( 'NONE',  ( -6.158143864569485777E-17, -2.736152283717910599E-16, 1.000000000000000000 ) ) ;
#6043=ORIENTED_EDGE ( 'NONE', *, *, #12796, .F. ) ;
#6046=DIRECTION ( 'NONE',  ( -0.9960067511297463483, 0.08927794634716618161, -4.818676322152979407E-17 ) ) ;
#6055=DIRECTION ( 'NONE',  ( -0.9960067511297463483, 0.08927794634716618161, -4.818676322152979407E-17 ) ) ;
#6057=ADVANCED_FACE ( 'NONE', ( #10822 ), #128, .T. ) ;
#6061=ORIENTED_EDGE ( 'NONE', *, *, #12991, .T. ) ;
#6068=DIRECTION ( 'NONE',  ( -6.158143864569485777E-17, -2.736152283717910599E-16, 1.000000000000000000 ) ) ;
#6078=CARTESIAN_POINT ( 'NONE',  ( 34.99999999999958789, 1.063887963769481123E-13, 12.50000000000000000 ) ) ;
#6090=CARTESIAN_POINT ( 'NONE',  ( 48.99302833075611119, 12.47878836808090064, -2.499999999999994671 ) ) ;
#6103=EDGE_CURVE ( 'NONE', #11376, #7898, #11703, .T. ) ;
#6105=DIRECTION ( 'NONE',  ( -6.158143864569485777E-17, -2.736152283717910599E-16, 1.000000000000000000 ) ) ;
#6106=AXIS2_PLACEMENT_3D ( 'NONE', #2651, #9166, #1009 ) ;
#6108=LINE ( 'NONE', #775, #11701 ) ;
#6119=CARTESIAN_POINT ( 'NONE',  ( 16.85679715600144135, -10.85606698379832125, 2.499999999999996003 ) ) ;
#6121=DIRECTION ( 'NONE',  ( -6.158143864569485777E-17, -2.736152283717910599E-16, 1.000000000000000000 ) ) ;
#6123=DIRECTION ( 'NONE',  ( -1.000000000000000000, 0.000000000000000000, 0.000000000000000000 ) ) ;
#6132=EDGE_CURVE ( 'NONE', #3347, #5217, #12844, .T. ) ;
#6134=AXIS2_PLACEMENT_3D ( 'NONE', #1397, #8905, #157 ) ;
#6141=DIRECTION ( 'NONE',  ( -0.6001121574638169642, 0.7999158696163758409, 1.927470528861191270E-16 ) ) ;
#6142=CIRCLE ( 'NONE', #10816, 18.74900000001875355 ) ;
#6146=CARTESIAN_POINT ( 'NONE',  ( 38.81043356982896597, -18.35771219435081392, -2.500000000000004441 ) ) ;
#6151=VERTEX_POINT ( 'NONE', #1206 ) ;
#6152=LINE ( 'NONE', #5090, #1689 ) ;
#6155=CARTESIAN_POINT ( 'NONE',  ( 43.63403238902020576, 20.33700654369049587, -2.499999999999992895 ) ) ;
#6162=AXIS2_PLACEMENT_3D ( 'NONE', #10011, #5512, #10768 ) ;
#6164=VECTOR ( 'NONE', #2273, 1000.000000000000000 ) ;
#6168=ORIENTED_EDGE ( 'NONE', *, *, #3163, .F. ) ;
#6171=DIRECTION ( 'NONE',  ( 0.4226182617407014397, -0.9063077870366489375, -0.000000000000000000 ) ) ;
#6178=EDGE_CURVE ( 'NONE', #10530, #4194, #4534, .T. ) ;
#6179=ORIENTED_EDGE ( 'NONE', *, *, #4650, .T. ) ;
#6185=CARTESIAN_POINT ( 'NONE',  ( 30.45476892764376231, 18.18971895053902443, -2.499999999999993783 ) ) ;
#6187=EDGE_LOOP ( 'NONE', ( #7303, #7001, #11986, #3267 ) ) ;
#6195=EDGE_CURVE ( 'NONE', #3082, #7032, #13769, .T. ) ;
#6202=EDGE_CURVE ( 'NONE', #750, #12212, #8768, .T. ) ;
#6203=ADVANCED_FACE ( 'NONE', ( #2458 ), #168, .T. ) ;
#6204=DIRECTION ( 'NONE',  ( 6.158143864569485777E-17, 2.736152283717910599E-16, -1.000000000000000000 ) ) ;
#6205=ORIENTED_EDGE ( 'NONE', *, *, #5303, .T. ) ;
#6206=CARTESIAN_POINT ( 'NONE',  ( 14.20591609908152009, -14.75994833063034761, -4.336808689942017736E-15 ) ) ;
#6232=ORIENTED_EDGE ( 'NONE', *, *, #6039, .T. ) ;
#6236=CARTESIAN_POINT ( 'NONE',  ( 23.44929957547844879, 14.76842309468663572, 2.500000000000003553 ) ) ;
#6239=CARTESIAN_POINT ( 'NONE',  ( 26.69171018101576465, -19.44228176112429551, -2.500000000000004441 ) ) ;
#6242=ORIENTED_EDGE ( 'NONE', *, *, #9996, .F. ) ;
#6243=VERTEX_POINT ( 'NONE', #9757 ) ;
#6247=EDGE_LOOP ( 'NONE', ( #13723, #7947, #2124, #10124 ) ) ;
#6250=DIRECTION ( 'NONE',  ( -6.158143864569485777E-17, -2.736152283717910599E-16, 1.000000000000000000 ) ) ;
#6255=FACE_OUTER_BOUND ( 'NONE', #1055, .T. ) ;
#6296=APPLICATION_CONTEXT ( 'automotive_design' ) ;
#6298=AXIS2_PLACEMENT_3D ( 'NONE', #6578, #5597, #4400 ) ;
#6299=AXIS2_PLACEMENT_3D ( 'NONE', #1607, #9114, #9042 ) ;
#6303=EDGE_CURVE ( 'NONE', #12930, #3310, #4919, .T. ) ;
#6304=DIRECTION ( 'NONE',  ( -6.158143864569485777E-17, -2.736152283717910599E-16, 1.000000000000000000 ) ) ;
#6309=ORIENTED_EDGE ( 'NONE', *, *, #12128, .F. ) ;
#6336=DIRECTION ( 'NONE',  ( -6.158143864569485777E-17, -2.736152283717910599E-16, 1.000000000000000000 ) ) ;
#6342=ORIENTED_EDGE ( 'NONE', *, *, #1724, .T. ) ;
#6347=CARTESIAN_POINT ( 'NONE',  ( 41.86252833142972918, 24.55922850786694056, 7.372574772901430151E-15 ) ) ;
#6355=CARTESIAN_POINT ( 'NONE',  ( 75.98647239440286683, -111.6214737678657087, 2.500000000000000000 ) ) ;
#6362=EDGE_CURVE ( 'NONE', #2145, #13485, #3646, .T. ) ;
#6363=PRESENTATION_STYLE_ASSIGNMENT (( #10828 ) ) ;
#6370=ADVANCED_FACE ( 'NONE', ( #6383 ), #7350, .T. ) ;
#6382=ORIENTED_EDGE ( 'NONE', *, *, #2173, .T. ) ;
#6383=FACE_OUTER_BOUND ( 'NONE', #4484, .T. ) ;
#6384=CARTESIAN_POINT ( 'NONE',  ( 32.61455173758670867, 25.38817907193537593, -2.499999999999992450 ) ) ;
#6393=ORIENTED_EDGE ( 'NONE', *, *, #708, .F. ) ;
#6397=EDGE_LOOP ( 'NONE', ( #5555, #11292, #6609, #7610 ) ) ;
#6408=CARTESIAN_POINT ( 'NONE',  ( 34.99999999999958789, 1.104930248025249758E-13, -2.499999999999997335 ) ) ;
#6412=LINE ( 'NONE', #9703, #5584 ) ;
#6414=DIRECTION ( 'NONE',  ( -6.158143864569485777E-17, -2.736152283717910599E-16, 1.000000000000000000 ) ) ;
#6418=DIRECTION ( 'NONE',  ( -6.158143864569485777E-17, -2.736152283717910599E-16, 1.000000000000000000 ) ) ;
#6420=ADVANCED_FACE ( 'NONE', ( #11509 ), #10391, .T. ) ;
#6431=ORIENTED_EDGE ( 'NONE', *, *, #6303, .T. ) ;
#6432=DIRECTION ( 'NONE',  ( 6.158143864569485777E-17, 2.736152283717910599E-16, -1.000000000000000000 ) ) ;
#6442=ORIENTED_EDGE ( 'NONE', *, *, #10554, .T. ) ;
#6445=ORIENTED_EDGE ( 'NONE', *, *, #8930, .F. ) ;
#6449=FACE_OUTER_BOUND ( 'NONE', #5116, .T. ) ;
#6451=ADVANCED_FACE ( 'NONE', ( #3083 ), #8283, .T. ) ;
#6453=DIRECTION ( 'NONE',  ( -6.158143864569485777E-17, -2.736152283717910599E-16, 1.000000000000000000 ) ) ;
#6455=DIRECTION ( 'NONE',  ( 0.9960067511297464593, -0.08927794634716622324, 6.802837160686558945E-17 ) ) ;
#6463=VERTEX_POINT ( 'NONE', #5188 ) ;
#6464=CARTESIAN_POINT ( 'NONE',  ( 34.66997162884352690, 21.14050806081579736, 2.500000000000005773 ) ) ;
#6467=CYLINDRICAL_SURFACE ( 'NONE', #5808, 9.000000000008999024 ) ;
#6468=LINE ( 'NONE', #8305, #7198 ) ;
#6475=AXIS2_PLACEMENT_3D ( 'NONE', #5206, #13804, #1007 ) ;
#6476=APPLICATION_CONTEXT ( 'automotive_design' ) ;
#6477=CYLINDRICAL_SURFACE ( 'NONE', #5828, 9.000000000008999024 ) ;
#6484=FACE_OUTER_BOUND ( 'NONE', #6187, .T. ) ;
#6501=FILL_AREA_STYLE ('',( #13896 ) ) ;
#6502=ORIENTED_EDGE ( 'NONE', *, *, #686, .F. ) ;
#6510=ADVANCED_FACE ( 'NONE', ( #3145 ), #10370, .F. ) ;
#6514=AXIS2_PLACEMENT_3D ( 'NONE', #9489, #1845, #2898 ) ;
#6515=EDGE_CURVE ( 'NONE', #7693, #11081, #13328, .T. ) ;
#6528=ORIENTED_EDGE ( 'NONE', *, *, #458, .F. ) ;
#6530=VERTEX_POINT ( 'NONE', #7209 ) ;
#6531=EDGE_CURVE ( 'NONE', #12400, #576, #8371, .T. ) ;
#6533=AXIS2_PLACEMENT_3D ( 'NONE', #9133, #5986, #12072 ) ;
#6535=DIRECTION ( 'NONE',  ( -6.158143864569485777E-17, -2.736152283717910599E-16, 1.000000000000000000 ) ) ;
#6547=VERTEX_POINT ( 'NONE', #12147 ) ;
#6548=AXIS2_PLACEMENT_3D ( 'NONE', #4436, #9998, #2339 ) ;
#6552=ORIENTED_EDGE ( 'NONE', *, *, #13831, .F. ) ;
#6555=VERTEX_POINT ( 'NONE', #11492 ) ;
#6563=AXIS2_PLACEMENT_3D ( 'NONE', #6919, #4832, #9108 ) ;
#6568=CARTESIAN_POINT ( 'NONE',  ( 21.34086416022640265, 21.53318388236929692, -2.499999999999994671 ) ) ;
#6576=LINE ( 'NONE', #2230, #10305 ) ;
#6578=CARTESIAN_POINT ( 'NONE',  ( 34.99999999999958789, 1.091249486606660213E-13, 2.500000000000000000 ) ) ;
#6579=AXIS2_PLACEMENT_3D ( 'NONE', #9031, #12110, #13343 ) ;
#6583=CARTESIAN_POINT ( 'NONE',  ( 53.56517978609545594, 2.618988451796029349, -2.499999999999997335 ) ) ;
#6599=CARTESIAN_POINT ( 'NONE',  ( 50.48962708925064646, 14.39101985375337556, -2.499999999999993783 ) ) ;
#6600=EDGE_CURVE ( 'NONE', #13800, #4911, #6142, .T. ) ;
#6609=ORIENTED_EDGE ( 'NONE', *, *, #2502, .T. ) ;
#6610=LINE ( 'NONE', #10944, #7199 ) ;
#6611=DIRECTION ( 'NONE',  ( -6.158143864569485777E-17, -2.736152283717910599E-16, 1.000000000000000000 ) ) ;
#6613=CIRCLE ( 'NONE', #5050, 25.50000000002549783 ) ;
#6614=CYLINDRICAL_SURFACE ( 'NONE', #9522, 9.000000000008999024 ) ;
#6631=CARTESIAN_POINT ( 'NONE',  ( 30.45476892764376231, 18.18971895053902443, -2.499999999999993783 ) ) ;
#6635=CYLINDRICAL_SURFACE ( 'NONE', #10176, 9.000000000008999024 ) ;
#6645=ORIENTED_EDGE ( 'NONE', *, *, #9518, .T. ) ;
#6651=DIRECTION ( 'NONE',  ( -6.158143864569485777E-17, -2.736152283717910599E-16, 1.000000000000000000 ) ) ;
#6656=DIRECTION ( 'NONE',  ( -6.158143864569485777E-17, -2.736152283717910599E-16, 1.000000000000000000 ) ) ;
#6657=ORIENTED_EDGE ( 'NONE', *, *, #8834, .T. ) ;
#6661=DIRECTION ( 'NONE',  ( 0.000000000000000000, 0.000000000000000000, 1.000000000000000000 ) ) ;
#6665=DIRECTION ( 'NONE',  ( 0.9960067511297463483, -0.08927794634716618161, 4.818676322152979407E-17 ) ) ;
#6669=CARTESIAN_POINT ( 'NONE',  ( 23.90723890023449627, -15.11541108221136476, 2.499999999999995115 ) ) ;
#6673=VECTOR ( 'NONE', #9885, 1000.000000000000000 ) ;
#6674=EDGE_CURVE ( 'NONE', #12816, #2145, #7267, .T. ) ;
#6677=EDGE_CURVE ( 'NONE', #3661, #425, #3911, .T. ) ;
#6678=FACE_OUTER_BOUND ( 'NONE', #5102, .T. ) ;
#6683=ORIENTED_EDGE ( 'NONE', *, *, #3318, .T. ) ;
#6695=FACE_OUTER_BOUND ( 'NONE', #9351, .T. ) ;
#6697=CIRCLE ( 'NONE', #8050, 25.50000000002549783 ) ;
#6715=ORIENTED_EDGE ( 'NONE', *, *, #10567, .T. ) ;
#6734=ORIENTED_EDGE ( 'NONE', *, *, #12370, .T. ) ;
#6747=DIRECTION ( 'NONE',  ( 0.9960067511297463483, -0.08927794634716618161, 4.818676322152979407E-17 ) ) ;
#6751=ORIENTED_EDGE ( 'NONE', *, *, #10419, .T. ) ;
#6753=CIRCLE ( 'NONE', #9452, 25.50000000002549783 ) ;
#6760=DIRECTION ( 'NONE',  ( -6.158143864569485777E-17, -2.736152283717910599E-16, 1.000000000000000000 ) ) ;
#6769=ADVANCED_FACE ( 'NONE', ( #8536 ), #4250, .T. ) ;
#6770=DIRECTION ( 'NONE',  ( 0.9960067511297463483, -0.08927794634716620936, 4.626175998653454121E-17 ) ) ;
#6772=DIRECTION ( 'NONE',  ( -0.3926913852462016186, -0.9196703082917373484, -2.891205793291787644E-16 ) ) ;
#6784=AXIS2_PLACEMENT_3D ( 'NONE', #1147, #5687, #7575 ) ;
#6792=VERTEX_POINT ( 'NONE', #203 ) ;
#6804=EDGE_CURVE ( 'NONE', #1659, #4720, #12114, .T. ) ;
#6805=ORIENTED_EDGE ( 'NONE', *, *, #3842, .F. ) ;
#6814=CARTESIAN_POINT ( 'NONE',  ( 34.99999999999958789, 1.104930248025249758E-13, -2.499999999999999112 ) ) ;
#6815=CARTESIAN_POINT ( 'NONE',  ( 40.87368016229836343, -22.78235879061915270, -2.500000000000000000 ) ) ;
#6819=CARTESIAN_POINT ( 'NONE',  ( 19.06870874253413461, 13.90050210118286245, -2.499999999999996447 ) ) ;
#6820=DIRECTION ( 'NONE',  ( -6.158143864569485777E-17, -2.736152283717910599E-16, 1.000000000000000000 ) ) ;
#6821=VECTOR ( 'NONE', #8119, 1000.000000000000000 ) ;
#6839=CIRCLE ( 'NONE', #132, 80.00000000000001421 ) ;
#6846=CIRCLE ( 'NONE', #5486, 9.000000000009002576 ) ;
#6851=EDGE_CURVE ( 'NONE', #11572, #3347, #4338, .T. ) ;
#6861=UNCERTAINTY_MEASURE_WITH_UNIT (LENGTH_MEASURE( 1.000000000000000082E-05 ), #155, 'distance_accuracy_value', 'NONE');
#6886=CARTESIAN_POINT ( 'NONE',  ( 43.29712336220986657, 19.44704974301885159, -2.499999999999993783 ) ) ;
#6892=VERTEX_POINT ( 'NONE', #8670 ) ;
#6902=AXIS2_PLACEMENT_3D ( 'NONE', #7080, #12419, #13213 ) ;
#6912=CIRCLE ( 'NONE', #8946, 25.50000000002549783 ) ;
#6919=CARTESIAN_POINT ( 'NONE',  ( 19.50211115783503857, -14.38212227840833179, -2.500000000000004441 ) ) ;
#6922=ORIENTED_EDGE ( 'NONE', *, *, #3182, .T. ) ;
#6925=VECTOR ( 'NONE', #4087, 1000.000000000000000 ) ;
#6926=DIRECTION ( 'NONE',  ( -6.158143864569485777E-17, -2.736152283717910599E-16, 1.000000000000000000 ) ) ;
#6934=CYLINDRICAL_SURFACE ( 'NONE', #12524, 9.000000000008999024 ) ;
#6950=CIRCLE ( 'NONE', #7398, 25.50000000002549783 ) ;
#6963=ORIENTED_EDGE ( 'NONE', *, *, #12271, .F. ) ;
#6967=ADVANCED_FACE ( 'NONE', ( #10977 ), #1378, .T. ) ;
#6969=LINE ( 'NONE', #3666, #1327 ) ;
#6973=CIRCLE ( 'NONE', #930, 25.50000000002549783 ) ;
#6974=DIRECTION ( 'NONE',  ( 0.9960067511297463483, -0.08927794634716618161, 4.818676322152979407E-17 ) ) ;
#6977=DIRECTION ( 'NONE',  ( 0.9960067511297464593, -0.08927794634716622324, 3.401418580343279473E-17 ) ) ;
#6981=DIRECTION ( 'NONE',  ( -0.9960067511297463483, 0.08927794634716619548, -4.626175998653453504E-17 ) ) ;
#6983=CARTESIAN_POINT ( 'NONE',  ( 34.99999999999958789, 1.104930248025249758E-13, -2.499999999999999112 ) ) ;
#6984=EDGE_CURVE ( 'NONE', #750, #3802, #5027, .T. ) ;
#6989=ORIENTED_EDGE ( 'NONE', *, *, #12483, .F. ) ;
#6996=DIRECTION ( 'NONE',  ( 6.158143864569485777E-17, 2.736152283717910599E-16, -1.000000000000000000 ) ) ;
#7001=ORIENTED_EDGE ( 'NONE', *, *, #1724, .F. ) ;
#7006=CARTESIAN_POINT ( 'NONE',  ( 34.99999999999958789, 1.104930248025249758E-13, -2.499999999999999112 ) ) ;
#7013=AXIS2_PLACEMENT_3D ( 'NONE', #2358, #10833, #5583 ) ;
#7020=ORIENTED_EDGE ( 'NONE', *, *, #5513, .F. ) ;
#7023=CARTESIAN_POINT ( 'NONE',  ( 16.85679715600144135, -10.85606698379831947, -2.500000000000003553 ) ) ;
#7025=CARTESIAN_POINT ( 'NONE',  ( 16.53267785980283477, 10.29504797295195750, -2.499999999999997335 ) ) ;
#7027=DIRECTION ( 'NONE',  ( 0.1928999275155752480, 0.9812184353977893014, 2.891205793291787644E-16 ) ) ;
#7032=VERTEX_POINT ( 'NONE', #9241 ) ;
#7042=DIRECTION ( 'NONE',  ( -6.158143864569485777E-17, -2.736152283717910599E-16, 1.000000000000000000 ) ) ;
#7043=ADVANCED_FACE ( 'NONE', ( #1096 ), #12954, .T. ) ;
#7045=CARTESIAN_POINT ( 'NONE',  ( 55.99165482216006495, 2.525950835318804266, -2.499999999999997335 ) ) ;
#7050=ORIENTED_EDGE ( 'NONE', *, *, #9673, .F. ) ;
#7067=EDGE_LOOP ( 'NONE', ( #2883, #6805, #116, #4718 ) ) ;
#7077=CARTESIAN_POINT ( 'NONE',  ( 52.85884796071297131, 5.708463060827147828, 2.500000000000002665 ) ) ;
#7080=CARTESIAN_POINT ( 'NONE',  ( 34.99999999999958789, 1.104930248025249758E-13, -2.499999999999997335 ) ) ;
#7093=CARTESIAN_POINT ( 'NONE',  ( 75.98647239440286683, -111.6214737678657087, 2.500000000000000000 ) ) ;
#7097=DIRECTION ( 'NONE',  ( -0.8735848310779960046, 0.4866719047884612293, 9.637352644305955116E-17 ) ) ;
#7107=CARTESIAN_POINT ( 'NONE',  ( 39.08445607832919677, 20.74481184150345214, 2.500000000000006217 ) ) ;
#7112=DIRECTION ( 'NONE',  ( -6.158143864569485777E-17, -2.736152283717910599E-16, 1.000000000000000000 ) ) ;
#7120=VERTEX_POINT ( 'NONE', #11949 ) ;
#7121=CYLINDRICAL_SURFACE ( 'NONE', #2469, 25.50000000002549783 ) ;
#7122=EDGE_CURVE ( 'NONE', #11079, #5471, #4082, .T. ) ;
#7124=ORIENTED_EDGE ( 'NONE', *, *, #704, .F. ) ;
#7139=AXIS2_PLACEMENT_3D ( 'NONE', #526, #3653, #8084 ) ;
#7149=DIRECTION ( 'NONE',  ( 0.9928035427100112553, 0.1197544386753605361, 9.637352644305958814E-17 ) ) ;
#7150=ORIENTED_EDGE ( 'NONE', *, *, #796, .F. ) ;
#7152=EDGE_LOOP ( 'NONE', ( #48, #1664, #2593, #11540 ) ) ;
#7156=ORIENTED_EDGE ( 'NONE', *, *, #12370, .F. ) ;
#7158=DIRECTION ( 'NONE',  ( -6.158143864569485777E-17, -2.736152283717910599E-16, 1.000000000000000000 ) ) ;
#7170=( GEOMETRIC_REPRESENTATION_CONTEXT ( 3 ) GLOBAL_UNCERTAINTY_ASSIGNED_CONTEXT ( ( #6861 ) ) GLOBAL_UNIT_ASSIGNED_CONTEXT ( ( #155, #12852, #1130 ) ) REPRESENTATION_CONTEXT ( 'NONE', 'WORKASPACE' ) );
#7174=VECTOR ( 'NONE', #10491, 1000.000000000000114 ) ;
#7190=DIRECTION ( 'NONE',  ( 0.9928035427100112553, 0.1197544386753605361, 9.637352644305958814E-17 ) ) ;
#7198=VECTOR ( 'NONE', #5277, 1000.000000000000000 ) ;
#7199=VECTOR ( 'NONE', #7792, 1000.000000000000000 ) ;
#7205=EDGE_CURVE ( 'NONE', #5202, #1244, #10507, .T. ) ;
#7206=VERTEX_POINT ( 'NONE', #9089 ) ;
#7209=CARTESIAN_POINT ( 'NONE',  ( 55.16425081158429577, -10.83695794929874090, 2.499999999999998224 ) ) ;
#7212=DIRECTION ( 'NONE',  ( -6.158143864569485777E-17, -2.736152283717910599E-16, 1.000000000000000000 ) ) ;
#7216=EDGE_LOOP ( 'NONE', ( #9305, #4570, #10195, #7745 ) ) ;
#7228=CARTESIAN_POINT ( 'NONE',  ( 34.99999999999958789, 1.063887963769481123E-13, 12.50000000000000000 ) ) ;
#7238=ORIENTED_EDGE ( 'NONE', *, *, #7464, .F. ) ;
#7239=AXIS2_PLACEMENT_3D ( 'NONE', #4637, #771, #2944 ) ;
#7246=CARTESIAN_POINT ( 'NONE',  ( 38.81043356982896597, -18.35771219435081392, -2.500000000000004441 ) ) ;
#7265=DIRECTION ( 'NONE',  ( -6.158143864569485777E-17, -2.736152283717910599E-16, 1.000000000000000000 ) ) ;
#7267=CIRCLE ( 'NONE', #13325, 18.74900000001875355 ) ;
#7281=EDGE_CURVE ( 'NONE', #7540, #3278, #8056, .T. ) ;
#7284=AXIS2_PLACEMENT_3D ( 'NONE', #10046, #9979, #9000 ) ;
#7290=EDGE_CURVE ( 'NONE', #11147, #13800, #5139, .T. ) ;
#7294=ORIENTED_EDGE ( 'NONE', *, *, #10894, .T. ) ;
#7299=FACE_OUTER_BOUND ( 'NONE', #8622, .T. ) ;
#7303=ORIENTED_EDGE ( 'NONE', *, *, #13423, .F. ) ;
#7308=ADVANCED_FACE ( 'NONE', ( #5209 ), #12665, .F. ) ;
#7325=DIRECTION ( 'NONE',  ( 6.158143864569485777E-17, 2.736152283717910599E-16, -1.000000000000000000 ) ) ;
#7326=CARTESIAN_POINT ( 'NONE',  ( 32.61455173758670867, 25.38817907193537593, 2.500000000000007105 ) ) ;
#7330=FACE_OUTER_BOUND ( 'NONE', #1025, .T. ) ;
#7335=DIRECTION ( 'NONE',  ( 0.9960067511297463483, -0.08927794634716620936, 4.626175998653454121E-17 ) ) ;
#7339=CARTESIAN_POINT ( 'NONE',  ( 23.18128365339294916, -22.59575057217061200, -2.500000000000006217 ) ) ;
#7340=VECTOR ( 'NONE', #844, 1000.000000000000000 ) ;
#7345=CARTESIAN_POINT ( 'NONE',  ( 38.24615002434714484, 18.46584715143433542, -2.499999999999993783 ) ) ;
#7350=CYLINDRICAL_SURFACE ( 'NONE', #4105, 9.000000000008999024 ) ;
#7351=EDGE_CURVE ( 'NONE', #11251, #3661, #945, .T. ) ;
#7355=DIRECTION ( 'NONE',  ( -0.2228746399763463781, 0.9748471135800803600, 2.544396799259399212E-16 ) ) ;
#7363=AXIS2_PLACEMENT_3D ( 'NONE', #4213, #1981, #12657 ) ;
#7367=CARTESIAN_POINT ( 'NONE',  ( 21.34086416022640265, 21.53318388236929692, 2.500000000000005329 ) ) ;
#7378=AXIS2_PLACEMENT_3D ( 'NONE', #7659, #6611, #13164 ) ;
#7379=CARTESIAN_POINT ( 'NONE',  ( 34.99999999999958789, 1.104930248025249758E-13, -2.499999999999999112 ) ) ;
#7394=CYLINDRICAL_SURFACE ( 'NONE', #11965, 25.50000000002549783 ) ;
#7398=AXIS2_PLACEMENT_3D ( 'NONE', #7379, #11667, #1991 ) ;
#7407=CIRCLE ( 'NONE', #4959, 18.74900000001875711 ) ;
#7410=CIRCLE ( 'NONE', #12126, 9.000000000008999024 ) ;
#7416=LINE ( 'NONE', #4057, #10690 ) ;
#7417=CARTESIAN_POINT ( 'NONE',  ( 23.44929957547844879, 14.76842309468663750, -2.499999999999996447 ) ) ;
#7426=DIRECTION ( 'NONE',  ( 0.01532218268402011502, -0.9998826084685129567, -2.891205793291787644E-16 ) ) ;
#7427=AXIS2_PLACEMENT_3D ( 'NONE', #7228, #789, #5192 ) ;
#7429=CYLINDRICAL_SURFACE ( 'NONE', #12134, 18.74900000001875000 ) ;
#7440=CYLINDRICAL_SURFACE ( 'NONE', #1024, 18.74900000001875000 ) ;
#7447=DIRECTION ( 'NONE',  ( -6.158143864569485777E-17, -2.736152283717910599E-16, 1.000000000000000000 ) ) ;
#7450=CARTESIAN_POINT ( 'NONE',  ( 34.99999999999958789, 1.091249486606660213E-13, 2.500000000000000000 ) ) ;
#7453=VECTOR ( 'NONE', #2445, 1000.000000000000000 ) ;
#7454=EDGE_LOOP ( 'NONE', ( #4160, #2306, #5571, #8365 ) ) ;
#7457=AXIS2_PLACEMENT_3D ( 'NONE', #8838, #3494, #5404 ) ;
#7462=EDGE_LOOP ( 'NONE', ( #5964, #2401, #12690, #2421 ) ) ;
#7463=CARTESIAN_POINT ( 'NONE',  ( 26.09988479906369463, 19.17858047941126642, -2.499999999999993783 ) ) ;
#7464=EDGE_CURVE ( 'NONE', #182, #12385, #7785, .T. ) ;
#7468=VECTOR ( 'NONE', #11933, 1000.000000000000000 ) ;
#7491=ADVANCED_FACE ( 'NONE', ( #11930 ), #172, .T. ) ;
#7498=CARTESIAN_POINT ( 'NONE',  ( 34.99999999999958789, 1.091249486606660213E-13, 2.500000000000000000 ) ) ;
#7502=ORIENTED_EDGE ( 'NONE', *, *, #5572, .F. ) ;
#7504=ORIENTED_EDGE ( 'NONE', *, *, #1401, .T. ) ;
#7505=VECTOR ( 'NONE', #2619, 1000.000000000000000 ) ;
#7524=DIRECTION ( 'NONE',  ( 0.9960067511297463483, -0.08927794634716618161, 4.818676322152979407E-17 ) ) ;
#7540=VERTEX_POINT ( 'NONE', #7093 ) ;
#7544=EDGE_CURVE ( 'NONE', #9863, #4263, #994, .T. ) ;
#7552=ORIENTED_EDGE ( 'NONE', *, *, #8130, .T. ) ;
#7554=EDGE_LOOP ( 'NONE', ( #3947, #3597, #2329, #6683 ) ) ;
#7561=AXIS2_PLACEMENT_3D ( 'NONE', #9410, #6121, #925 ) ;
#7567=EDGE_CURVE ( 'NONE', #3229, #12269, #9413, .T. ) ;
#7573=CARTESIAN_POINT ( 'NONE',  ( 47.16901142695026294, 17.29003067336574517, 2.500000000000005773 ) ) ;
#7575=DIRECTION ( 'NONE',  ( -0.2228746399763463781, 0.9748471135800803600, 2.544396799259399212E-16 ) ) ;
#7587=DIRECTION ( 'NONE',  ( -6.158143864569485777E-17, -2.736152283717910599E-16, 1.000000000000000000 ) ) ;
#7593=DIRECTION ( 'NONE',  ( 1.000000000000000000, 0.000000000000000000, 0.000000000000000000 ) ) ;
#7594=ORIENTED_EDGE ( 'NONE', *, *, #6677, .T. ) ;
#7595=LINE ( 'NONE', #254, #6164 ) ;
#7602=DIRECTION ( 'NONE',  ( -6.158143864569485777E-17, -2.736152283717910599E-16, 1.000000000000000000 ) ) ;
#7610=ORIENTED_EDGE ( 'NONE', *, *, #5303, .F. ) ;
#7616=DIRECTION ( 'NONE',  ( -6.158143864569485777E-17, -2.736152283717910599E-16, 1.000000000000000000 ) ) ;
#7632=CYLINDRICAL_SURFACE ( 'NONE', #4200, 9.000000000008999024 ) ;
#7645=DIRECTION ( 'NONE',  ( -6.158143864569485777E-17, -2.736152283717910599E-16, 1.000000000000000000 ) ) ;
#7646=ORIENTED_EDGE ( 'NONE', *, *, #10066, .T. ) ;
#7652=DIRECTION ( 'NONE',  ( -6.158143864569485777E-17, -2.736152283717910599E-16, 1.000000000000000000 ) ) ;
#7656=DIRECTION ( 'NONE',  ( 0.9960067511297464593, -0.08927794634716622324, 3.401418580343279473E-17 ) ) ;
#7659=CARTESIAN_POINT ( 'NONE',  ( 53.14943414785363984, 10.84564612680554241, -2.499999999999994671 ) ) ;
#7667=CARTESIAN_POINT ( 'NONE',  ( 35.08961652778860696, 18.74878582411816197, -2.499999999999993783 ) ) ;
#7676=AXIS2_PLACEMENT_3D ( 'NONE', #6119, #1902, #7426 ) ;
#7677=ORIENTED_EDGE ( 'NONE', *, *, #9461, .F. ) ;
#7682=DIRECTION ( 'NONE',  ( -6.158143864569485777E-17, -2.736152283717910599E-16, 1.000000000000000000 ) ) ;
#7685=UNCERTAINTY_MEASURE_WITH_UNIT (LENGTH_MEASURE( 1.000000000000000082E-05 ), #8533, 'distance_accuracy_value', 'NONE');
#7693=VERTEX_POINT ( 'NONE', #10913 ) ;
#7695=MANIFOLD_SOLID_BREP ( 'Join1', #10288 ) ;
#7696=LINE ( 'NONE', #11979, #6673 ) ;
#7710=CARTESIAN_POINT ( 'NONE',  ( 16.34455450841069890, -1.870656171256065425, -2.500000000000000888 ) ) ;
#7711=ORIENTED_EDGE ( 'NONE', *, *, #7281, .F. ) ;
#7713=DIRECTION ( 'NONE',  ( -6.158143864569485777E-17, -2.736152283717910599E-16, 1.000000000000000000 ) ) ;
#7716=AXIS2_PLACEMENT_3D ( 'NONE', #1481, #10041, #8318 ) ;
#7721=CIRCLE ( 'NONE', #9529, 25.50000000002549783 ) ;
#7723=VERTEX_POINT ( 'NONE', #7765 ) ;
#7740=CIRCLE ( 'NONE', #3260, 25.50000000002549783 ) ;
#7742=DIRECTION ( 'NONE',  ( -6.158143864569485777E-17, -2.736152283717910599E-16, 1.000000000000000000 ) ) ;
#7743=ADVANCED_FACE ( 'NONE', ( #10024 ), #9956, .T. ) ;
#7744=VERTEX_POINT ( 'NONE', #1611 ) ;
#7745=ORIENTED_EDGE ( 'NONE', *, *, #517, .T. ) ;
#7753=CARTESIAN_POINT ( 'NONE',  ( 13.94188849117746010, 1.893657697999893808, -2.500000000000000000 ) ) ;
#7764=CYLINDRICAL_SURFACE ( 'NONE', #12514, 25.50000000002549783 ) ;
#7765=CARTESIAN_POINT ( 'NONE',  ( 53.02537423504344360, -5.158573900538658386, 2.499999999999999556 ) ) ;
#7767=LINE ( 'NONE', #12054, #7453 ) ;
#7776=LINE ( 'NONE', #5685, #11421 ) ;
#7785=LINE ( 'NONE', #9762, #4 ) ;
#7791=CIRCLE ( 'NONE', #1535, 9.000000000008999024 ) ;
#7792=DIRECTION ( 'NONE',  ( -6.158143864569485777E-17, -2.736152283717910599E-16, 1.000000000000000000 ) ) ;
#7794=EDGE_CURVE ( 'NONE', #13136, #7032, #13284, .T. ) ;
#7801=ORIENTED_EDGE ( 'NONE', *, *, #4212, .T. ) ;
#7802=DIRECTION ( 'NONE',  ( -6.158143864569485777E-17, -2.736152283717910599E-16, 1.000000000000000000 ) ) ;
#7803=CIRCLE ( 'NONE', #442, 9.000000000008999024 ) ;
#7812=FACE_OUTER_BOUND ( 'NONE', #5916, .T. ) ;
#7817=VECTOR ( 'NONE', #9688, 1000.000000000000000 ) ;
#7818=ORIENTED_EDGE ( 'NONE', *, *, #12271, .T. ) ;
#7834=ORIENTED_EDGE ( 'NONE', *, *, #9693, .T. ) ;
#7836=EDGE_LOOP ( 'NONE', ( #11817, #10242, #10340, #12511 ) ) ;
#7850=DIRECTION ( 'NONE',  ( -6.158143864569485777E-17, -2.736152283717910599E-16, 1.000000000000000000 ) ) ;
#7851=ORIENTED_EDGE ( 'NONE', *, *, #2158, .T. ) ;
#7858=ORIENTED_EDGE ( 'NONE', *, *, #7290, .F. ) ;
#7864=CIRCLE ( 'NONE', #3608, 9.000000000008999024 ) ;
#7866=FACE_OUTER_BOUND ( 'NONE', #5854, .T. ) ;
#7878=DIRECTION ( 'NONE',  ( -6.158143864569485777E-17, -2.736152283717910599E-16, 1.000000000000000000 ) ) ;
#7879=CYLINDRICAL_SURFACE ( 'NONE', #4034, 25.50000000002549783 ) ;
#7895=DIRECTION ( 'NONE',  ( 0.08715574274765883200, -0.9961946980917454342, -0.000000000000000000 ) ) ;
#7898=VERTEX_POINT ( 'NONE', #9325 ) ;
#7901=EDGE_CURVE ( 'NONE', #6530, #7206, #4709, .T. ) ;
#7907=CIRCLE ( 'NONE', #971, 25.50000000002549783 ) ;
#7918=AXIS2_PLACEMENT_3D ( 'NONE', #13212, #10917, #220 ) ;
#7931=VERTEX_POINT ( 'NONE', #6236 ) ;
#7947=ORIENTED_EDGE ( 'NONE', *, *, #3429, .T. ) ;
#7953=VECTOR ( 'NONE', #12310, 1000.000000000000000 ) ;
#7956=VERTEX_POINT ( 'NONE', #7077 ) ;
#7958=ADVANCED_FACE ( 'NONE', ( #12486 ), #12563, .T. ) ;
#7966=DIRECTION ( 'NONE',  ( -1.000000000000000000, 0.000000000000000000, 0.000000000000000000 ) ) ;
#7974=VECTOR ( 'NONE', #11448, 1000.000000000000000 ) ;
#7977=EDGE_CURVE ( 'NONE', #5594, #11832, #13712, .T. ) ;
#7984=AXIS2_PLACEMENT_3D ( 'NONE', #11984, #6656, #1322 ) ;
#7992=ORIENTED_EDGE ( 'NONE', *, *, #4024, .F. ) ;
#7997=EDGE_CURVE ( 'NONE', #2860, #7931, #8466, .T. ) ;
#8021=VERTEX_POINT ( 'NONE', #9021 ) ;
#8027=FACE_OUTER_BOUND ( 'NONE', #25, .T. ) ;
#8046=CARTESIAN_POINT ( 'NONE',  ( 17.38503225228318883, -6.421675190136373779, -2.500000000000002665 ) ) ;
#8050=AXIS2_PLACEMENT_3D ( 'NONE', #4554, #5402, #10925 ) ;
#8054=CARTESIAN_POINT ( 'NONE',  ( 16.53267785980283477, 10.29504797295195573, 2.500000000000001776 ) ) ;
#8056=CIRCLE ( 'NONE', #10733, 80.00000000000001421 ) ;
#8059=CIRCLE ( 'NONE', #13702, 9.000000000008999024 ) ;
#8084=DIRECTION ( 'NONE',  ( 0.9960067511297464593, -0.08927794634716622324, 3.401418580343279473E-17 ) ) ;
#8088=FACE_OUTER_BOUND ( 'NONE', #1865, .T. ) ;
#8119=DIRECTION ( 'NONE',  ( -6.158143864569485777E-17, -2.736152283717910599E-16, 1.000000000000000000 ) ) ;
#8129=CIRCLE ( 'NONE', #5208, 9.000000000009000800 ) ;
#8130=EDGE_CURVE ( 'NONE', #12373, #6030, #2475, .T. ) ;
#8193=AXIS2_PLACEMENT_3D ( 'NONE', #1409, #10931, #382 ) ;
#8202=AXIS2_PLACEMENT_3D ( 'NONE', #946, #6336, #12523 ) ;
#8211=AXIS2_PLACEMENT_3D ( 'NONE', #5098, #13759, #9454 ) ;
#8235=CYLINDRICAL_SURFACE ( 'NONE', #8202, 9.000000000008999024 ) ;
#8246=ORIENTED_EDGE ( 'NONE', *, *, #8380, .F. ) ;
#8248=EDGE_CURVE ( 'NONE', #988, #5397, #6950, .T. ) ;
#8257=AXIS2_PLACEMENT_3D ( 'NONE', #6239, #1751, #7149 ) ;
#8278=LINE ( 'NONE', #6185, #12194 ) ;
#8283=CYLINDRICAL_SURFACE ( 'NONE', #11282, 9.000000000008999024 ) ;
#8295=FACE_BOUND ( 'NONE', #5735, .T. ) ;
#8296=VERTEX_POINT ( 'NONE', #3238 ) ;
#8305=CARTESIAN_POINT ( 'NONE',  ( 10.29982004912477578, -6.336490384724132952, -1.734723475976807094E-15 ) ) ;
#8306=DIRECTION ( 'NONE',  ( 0.9960067511297463483, -0.08927794634716619548, 0.000000000000000000 ) ) ;
#8314=VERTEX_POINT ( 'NONE', #5144 ) ;
#8318=DIRECTION ( 'NONE',  ( -0.9960067511297463483, 0.08927794634716618161, -4.818676322152979407E-17 ) ) ;
#8325=EDGE_CURVE ( 'NONE', #576, #5704, #1144, .T. ) ;
#8353=CARTESIAN_POINT ( 'NONE',  ( 30.29366116764611760, 20.61262658154624816, 2.500000000000005329 ) ) ;
#8355=DIRECTION ( 'NONE',  ( 0.000000000000000000, 0.000000000000000000, -1.000000000000000000 ) ) ;
#8359=ORIENTED_EDGE ( 'NONE', *, *, #3093, .T. ) ;
#8365=ORIENTED_EDGE ( 'NONE', *, *, #11757, .T. ) ;
#8366=FACE_OUTER_BOUND ( 'NONE', #1632, .T. ) ;
#8371=CIRCLE ( 'NONE', #86, 9.000000000009000800 ) ;
#8372=DIRECTION ( 'NONE',  ( 0.9960067511297464593, -0.08927794634716622324, 3.401418580343279473E-17 ) ) ;
#8375=ORIENTED_EDGE ( 'NONE', *, *, #10885, .T. ) ;
#8376=CARTESIAN_POINT ( 'NONE',  ( 47.69307742500824787, -16.90904448151677286, -2.500000000000002665 ) ) ;
#8380=EDGE_CURVE ( 'NONE', #11850, #6243, #13510, .T. ) ;
#8385=DIRECTION ( 'NONE',  ( -6.158143864569485777E-17, -2.736152283717910599E-16, 1.000000000000000000 ) ) ;
#8389=DIRECTION ( 'NONE',  ( -6.158143864569485777E-17, -2.736152283717910599E-16, 1.000000000000000000 ) ) ;
#8401=CIRCLE ( 'NONE', #4143, 18.74900000001875000 ) ;
#8406=DIRECTION ( 'NONE',  ( 0.5753203450992270263, 0.8179281756455796248, 2.409338161076488717E-16 ) ) ;
#8415=CARTESIAN_POINT ( 'NONE',  ( 33.39358510189354945, -25.44935030951552690, -2.500000000000006217 ) ) ;
#8422=LINE ( 'NONE', #856, #2656 ) ;
#8425=CARTESIAN_POINT ( 'NONE',  ( 14.53672965213156942, 15.21527412409548674, 2.500000000000003109 ) ) ;
#8428=CARTESIAN_POINT ( 'NONE',  ( 34.99999999999958789, 1.063887963769481123E-13, 12.50000000000000000 ) ) ;
#8431=EDGE_CURVE ( 'NONE', #6547, #3108, #7407, .T. ) ;
#8441=AXIS2_PLACEMENT_3D ( 'NONE', #66, #7682, #1180 ) ;
#8445=DIRECTION ( 'NONE',  ( 0.9960067511297463483, -0.08927794634716618161, 4.818676322152979407E-17 ) ) ;
#8456=CARTESIAN_POINT ( 'NONE',  ( 14.99223790936468603, -6.835163196276449860, -2.500000000000002665 ) ) ;
#8466=LINE ( 'NONE', #7417, #5163 ) ;
#8491=CARTESIAN_POINT ( 'NONE',  ( 62.16766351966359849, -73.17985663200910551, -2.500000000000000000 ) ) ;
#8493=EDGE_CURVE ( 'NONE', #11251, #11452, #3989, .T. ) ;
#8497=DIRECTION ( 'NONE',  ( -0.9960067511297463483, 0.08927794634716618161, -4.818676322152979407E-17 ) ) ;
#8509=ORIENTED_EDGE ( 'NONE', *, *, #124, .F. ) ;
#8511=CARTESIAN_POINT ( 'NONE',  ( 31.28009342530033265, 25.22721338310705264, 2.500000000000006661 ) ) ;
#8512=MECHANICAL_DESIGN_GEOMETRIC_PRESENTATION_REPRESENTATION('',(#12331),#7170);
#8517=ORIENTED_EDGE ( 'NONE', *, *, #5751, .F. ) ;
#8526=CARTESIAN_POINT ( 'NONE',  ( 34.99999999999958789, 1.104930248025249758E-13, -2.499999999999999112 ) ) ;
#8527=LINE ( 'NONE', #4174, #11829 ) ;
#8528=ADVANCED_FACE ( 'NONE', ( #10121 ), #730, .T. ) ;
#8531=CIRCLE ( 'NONE', #1606, 9.000000000008999024 ) ;
#8532=VECTOR ( 'NONE', #3380, 1000.000000000000000 ) ;
#8533=( LENGTH_UNIT ( ) NAMED_UNIT ( * ) SI_UNIT ( .MILLI., .METRE. ) );
#8534=ORIENTED_EDGE ( 'NONE', *, *, #1984, .T. ) ;
#8536=FACE_OUTER_BOUND ( 'NONE', #956, .T. ) ;
#8542=CIRCLE ( 'NONE', #2951, 9.000000000008999024 ) ;
#8548=VECTOR ( 'NONE', #5214, 1000.000000000000000 ) ;
#8550=PRESENTATION_STYLE_ASSIGNMENT (( #8822 ) ) ;
#8565=LINE ( 'NONE', #95, #5813 ) ;
#8568=DIRECTION ( 'NONE',  ( -6.158143864569485777E-17, -2.736152283717910599E-16, 1.000000000000000000 ) ) ;
#8579=CARTESIAN_POINT ( 'NONE',  ( 56.05919550416194141, -1.881564379087037553, -2.499999999999998224 ) ) ;
#8580=AXIS2_PLACEMENT_3D ( 'NONE', #11711, #6453, #13477 ) ;
#8585=ORIENTED_EDGE ( 'NONE', *, *, #5395, .F. ) ;
#8617=LINE ( 'NONE', #6583, #3884 ) ;
#8622=EDGE_LOOP ( 'NONE', ( #8534, #3011, #6309, #13645 ) ) ;
#8640=LINE ( 'NONE', #9697, #7468 ) ;
#8641=EDGE_CURVE ( 'NONE', #7744, #12738, #13207, .T. ) ;
#8651=CARTESIAN_POINT ( 'NONE',  ( 58.70736094381068426, -9.392073098158828515, -8.673617379884035472E-16 ) ) ;
#8659=ADVANCED_FACE ( 'NONE', ( #3560 ), #6934, .T. ) ;
#8663=AXIS2_PLACEMENT_3D ( 'NONE', #4875, #2634, #9091 ) ;
#8670=CARTESIAN_POINT ( 'NONE',  ( 18.71826692230518674, -9.296782722394514309, -2.500000000000002665 ) ) ;
#8676=VERTEX_POINT ( 'NONE', #12566 ) ;
#8691=ORIENTED_EDGE ( 'NONE', *, *, #4212, .F. ) ;
#8699=LINE ( 'NONE', #3369, #671 ) ;
#8700=FACE_OUTER_BOUND ( 'NONE', #4913, .T. ) ;
#8701=DIRECTION ( 'NONE',  ( 0.000000000000000000, 0.000000000000000000, -1.000000000000000000 ) ) ;
#8703=AXIS2_PLACEMENT_3D ( 'NONE', #1915, #6204, #10465 ) ;
#8709=CARTESIAN_POINT ( 'NONE',  ( 60.47785218637952198, 1.062566689801825781, 2.168404344971008868E-15 ) ) ;
#8714=CARTESIAN_POINT ( 'NONE',  ( 14.79219767565756527, 6.218900627562690353, 2.500000000000000444 ) ) ;
#8720=CARTESIAN_POINT ( 'NONE',  ( 48.99302833075611119, 12.47878836808089886, 2.500000000000004441 ) ) ;
#8742=EDGE_CURVE ( 'NONE', #6892, #4054, #13572, .T. ) ;
#8745=ORIENTED_EDGE ( 'NONE', *, *, #3442, .F. ) ;
#8748=EDGE_CURVE ( 'NONE', #8021, #6030, #10312, .T. ) ;
#8752=CARTESIAN_POINT ( 'NONE',  ( 31.01425004688410070, -18.32044754671509423, -2.500000000000004441 ) ) ;
#8755=EDGE_CURVE ( 'NONE', #10021, #6151, #9810, .T. ) ;
#8767=ORIENTED_EDGE ( 'NONE', *, *, #6103, .F. ) ;
#8768=LINE ( 'NONE', #11009, #4097 ) ;
#8769=DIRECTION ( 'NONE',  ( 0.9960067511297464593, -0.08927794634716622324, 3.401418580343279473E-17 ) ) ;
#8789=ORIENTED_EDGE ( 'NONE', *, *, #6178, .T. ) ;
#8798=CARTESIAN_POINT ( 'NONE',  ( 82.09155748149851206, -71.43674177705591433, 2.500000000000000000 ) ) ;
#8803=CIRCLE ( 'NONE', #2780, 25.50000000002549783 ) ;
#8806=ORIENTED_EDGE ( 'NONE', *, *, #1291, .F. ) ;
#8810=CARTESIAN_POINT ( 'NONE',  ( 34.99999999999958789, 1.104930248025249758E-13, -2.499999999999999112 ) ) ;
#8813=ORIENTED_EDGE ( 'NONE', *, *, #4117, .F. ) ;
#8816=EDGE_CURVE ( 'NONE', #3113, #3156, #1979, .T. ) ;
#8821=CARTESIAN_POINT ( 'NONE',  ( 9.857979974958242408, 4.257796268226277547, 2.499999999999999556 ) ) ;
#8822=SURFACE_STYLE_USAGE ( .BOTH. , #4544 ) ;
#8827=ORIENTED_EDGE ( 'NONE', *, *, #10894, .F. ) ;
#8834=EDGE_CURVE ( 'NONE', #8676, #5851, #1756, .T. ) ;
#8836=DIRECTION ( 'NONE',  ( -6.158143864569485777E-17, -2.736152283717910599E-16, 1.000000000000000000 ) ) ;
#8838=CARTESIAN_POINT ( 'NONE',  ( 26.09988479906369463, 19.17858047941126642, -2.499999999999993783 ) ) ;
#8858=CARTESIAN_POINT ( 'NONE',  ( 34.99999999999958789, 1.104930248025249758E-13, -2.499999999999999112 ) ) ;
#8859=CARTESIAN_POINT ( 'NONE',  ( 34.99999999999958789, 1.091249486606660213E-13, 2.500000000000000000 ) ) ;
#8883=ORIENTED_EDGE ( 'NONE', *, *, #5674, .T. ) ;
#8885=ORIENTED_EDGE ( 'NONE', *, *, #11581, .F. ) ;
#8893=CARTESIAN_POINT ( 'NONE',  ( 16.34455450841069890, -1.870656171256065425, -2.500000000000000888 ) ) ;
#8905=DIRECTION ( 'NONE',  ( -6.158143864569485777E-17, -2.736152283717910599E-16, 1.000000000000000000 ) ) ;
#8908=ORIENTED_EDGE ( 'NONE', *, *, #1538, .T. ) ;
#8910=ORIENTED_EDGE ( 'NONE', *, *, #12889, .F. ) ;
#8911=ORIENTED_EDGE ( 'NONE', *, *, #17, .T. ) ;
#8918=AXIS2_PLACEMENT_3D ( 'NONE', #8353, #992, #5257 ) ;
#8926=DIRECTION ( 'NONE',  ( -6.158143864569485777E-17, -2.736152283717910599E-16, 1.000000000000000000 ) ) ;
#8930=EDGE_CURVE ( 'NONE', #11500, #4518, #6912, .T. ) ;
#8932=ORIENTED_EDGE ( 'NONE', *, *, #11387, .F. ) ;
#8936=CIRCLE ( 'NONE', #4674, 9.000000000008999024 ) ;
#8939=DIRECTION ( 'NONE',  ( 0.9960067511297463483, -0.08927794634716620936, 4.626175998653454121E-17 ) ) ;
#8940=DIRECTION ( 'NONE',  ( 0.7533101279583153120, -0.6576654553155629745, -1.387852799596036359E-16 ) ) ;
#8946=AXIS2_PLACEMENT_3D ( 'NONE', #3277, #11899, #2291 ) ;
#8950=DIRECTION ( 'NONE',  ( 0.01532218268401990685, -0.9998826084685129567, -2.775705599192072226E-16 ) ) ;
#8952=CARTESIAN_POINT ( 'NONE',  ( 34.66997162884352690, 21.14050806081579736, -2.499999999999992895 ) ) ;
#8959=ORIENTED_EDGE ( 'NONE', *, *, #456, .T. ) ;
#8973=AXIS2_PLACEMENT_3D ( 'NONE', #13492, #11276, #13557 ) ;
#8977=LINE ( 'NONE', #4843, #12964 ) ;
#8981=AXIS2_PLACEMENT_3D ( 'NONE', #10412, #13744, #8372 ) ;
#9000=DIRECTION ( 'NONE',  ( -0.9462100554738961389, -0.3235529800822217195, -1.387852799596036113E-16 ) ) ;
#9013=DIRECTION ( 'NONE',  ( 1.000000000000000000, 0.000000000000000000, 0.000000000000000000 ) ) ;
#9021=CARTESIAN_POINT ( 'NONE',  ( 60.49844721164429728, -0.2814068163155458158, -2.499999999999997335 ) ) ;
#9031=CARTESIAN_POINT ( 'NONE',  ( 76.84607712649204814, -99.92541302764922762, 2.500000000000000000 ) ) ;
#9038=ORIENTED_EDGE ( 'NONE', *, *, #1538, .F. ) ;
#9042=DIRECTION ( 'NONE',  ( -0.7328050451781167318, -0.6804386568688601811, -2.313087999326727184E-16 ) ) ;
#9050=CYLINDRICAL_SURFACE ( 'NONE', #815, 2.500000000000000444 ) ;
#9058=VERTEX_POINT ( 'NONE', #1804 ) ;
#9061=ORIENTED_EDGE ( 'NONE', *, *, #5450, .T. ) ;
#9067=FACE_OUTER_BOUND ( 'NONE', #2876, .T. ) ;
#9070=CARTESIAN_POINT ( 'NONE',  ( 34.99999999999958789, 1.063887963769481123E-13, 12.50000000000000000 ) ) ;
#9078=DIRECTION ( 'NONE',  ( -6.158143864569485777E-17, -2.736152283717910599E-16, 1.000000000000000000 ) ) ;
#9080=DIRECTION ( 'NONE',  ( -0.9960067511297463483, 0.08927794634716618161, -4.818676322152979407E-17 ) ) ;
#9089=CARTESIAN_POINT ( 'NONE',  ( 58.17953216333035726, -10.62823074130461620, 2.499999999999998668 ) ) ;
#9091=DIRECTION ( 'NONE',  ( 0.7533101279583152010, -0.6576654553155629745, -1.445602896645893576E-16 ) ) ;
#9105=FACE_OUTER_BOUND ( 'NONE', #5037, .T. ) ;
#9108=DIRECTION ( 'NONE',  ( 0.9556796851544554494, -0.2944084567112178474, 0.000000000000000000 ) ) ;
#9110=ADVANCED_FACE ( 'NONE', ( #11551 ), #13763, .T. ) ;
#9114=DIRECTION ( 'NONE',  ( -6.158143864569485777E-17, -2.736152283717910599E-16, 1.000000000000000000 ) ) ;
#9120=CARTESIAN_POINT ( 'NONE',  ( 18.44105126153190710, 8.793532718851094998, -2.499999999999998224 ) ) ;
#9133=CARTESIAN_POINT ( 'NONE',  ( 34.99999999999958789, 1.104930248025249758E-13, -2.499999999999999112 ) ) ;
#9135=DIRECTION ( 'NONE',  ( 0.9960067511297464593, -0.08927794634716622324, 6.802837160686558945E-17 ) ) ;
#9154=CYLINDRICAL_SURFACE ( 'NONE', #9935, 9.000000000008999024 ) ;
#9158=ORIENTED_EDGE ( 'NONE', *, *, #3809, .T. ) ;
#9162=ORIENTED_EDGE ( 'NONE', *, *, #4890, .F. ) ;
#9166=DIRECTION ( 'NONE',  ( -6.158143864569485777E-17, -2.736152283717910599E-16, 1.000000000000000000 ) ) ;
#9167=DIRECTION ( 'NONE',  ( -6.158143864569485777E-17, -2.736152283717910599E-16, 1.000000000000000000 ) ) ;
#9172=VERTEX_POINT ( 'NONE', #9313 ) ;
#9203=CARTESIAN_POINT ( 'NONE',  ( 21.12690199240172007, 12.61198448588842425, -2.499999999999996447 ) ) ;
#9206=FACE_OUTER_BOUND ( 'NONE', #9667, .T. ) ;
#9210=VERTEX_POINT ( 'NONE', #5301 ) ;
#9213=ORIENTED_EDGE ( 'NONE', *, *, #2234, .T. ) ;
#9215=AXIS2_PLACEMENT_3D ( 'NONE', #3375, #2187, #390 ) ;
#9216=ADVANCED_FACE ( 'NONE', ( #3394 ), #13828, .T. ) ;
#9219=CIRCLE ( 'NONE', #13275, 9.000000000008999024 ) ;
#9241=CARTESIAN_POINT ( 'NONE',  ( 43.63403238902020576, 20.33700654369049587, 2.500000000000006217 ) ) ;
#9245=DIRECTION ( 'NONE',  ( -1.000000000000000000, 0.000000000000000000, 0.000000000000000000 ) ) ;
#9247=EDGE_LOOP ( 'NONE', ( #1389, #6734, #13015, #13863 ) ) ;
#9258=EDGE_CURVE ( 'NONE', #11079, #752, #8527, .T. ) ;
#9259=VECTOR ( 'NONE', #10849, 1000.000000000000000 ) ;
#9260=ORIENTED_EDGE ( 'NONE', *, *, #11581, .T. ) ;
#9268=CYLINDRICAL_SURFACE ( 'NONE', #11391, 18.74900000001875000 ) ;
#9280=VECTOR ( 'NONE', #1056, 1000.000000000000000 ) ;
#9283=DIRECTION ( 'NONE',  ( 0.4206864060305147146, -0.9072061219927526343, -2.313087999326727677E-16 ) ) ;
#9290=CARTESIAN_POINT ( 'NONE',  ( 27.45605056404223987, 17.16431845161425684, 2.500000000000004441 ) ) ;
#9302=AXIS2_PLACEMENT_3D ( 'NONE', #4653, #4504, #5551 ) ;
#9305=ORIENTED_EDGE ( 'NONE', *, *, #12889, .T. ) ;
#9313=CARTESIAN_POINT ( 'NONE',  ( 57.84299132690245671, 11.33347904398042871, 2.500000000000004441 ) ) ;
#9325=CARTESIAN_POINT ( 'NONE',  ( 32.50998312217522113, 0.2231948658680255604, 2.500000000000000000 ) ) ;
#9330=ORIENTED_EDGE ( 'NONE', *, *, #10693, .F. ) ;
#9337=DIRECTION ( 'NONE',  ( -6.158143864569485777E-17, -2.736152283717910599E-16, 1.000000000000000000 ) ) ;
#9351=EDGE_LOOP ( 'NONE', ( #9061, #2178, #13246, #10893 ) ) ;
#9352=DIRECTION ( 'NONE',  ( -6.158143864569485777E-17, -2.736152283717910599E-16, 1.000000000000000000 ) ) ;
#9357=ADVANCED_FACE ( 'NONE', ( #6695 ), #1584, .T. ) ;
#9359=DIRECTION ( 'NONE',  ( 0.9556796851544554494, -0.2944084567112178474, 0.000000000000000000 ) ) ;
#9363=EDGE_CURVE ( 'NONE', #11081, #1977, #7803, .T. ) ;
#9372=ORIENTED_EDGE ( 'NONE', *, *, #9523, .T. ) ;
#9394=CIRCLE ( 'NONE', #3329, 18.74900000001874645 ) ;
#9399=FACE_OUTER_BOUND ( 'NONE', #4232, .T. ) ;
#9410=CARTESIAN_POINT ( 'NONE',  ( 50.92330601230504783, -13.90964864522661415, -2.500000000000001776 ) ) ;
#9412=CARTESIAN_POINT ( 'NONE',  ( 60.47785218637952198, 1.062566689801823117, -2.499999999999997335 ) ) ;
#9413=CIRCLE ( 'NONE', #10522, 9.000000000008999024 ) ;
#9418=ADVANCED_FACE ( 'NONE', ( #4515 ), #3463, .F. ) ;
#9441=CIRCLE ( 'NONE', #6299, 18.74900000001875000 ) ;
#9452=AXIS2_PLACEMENT_3D ( 'NONE', #1108, #4738, #11987 ) ;
#9453=CARTESIAN_POINT ( 'NONE',  ( 76.84607712649204814, -99.92541302764922762, -2.500000000000000000 ) ) ;
#9454=DIRECTION ( 'NONE',  ( 0.9960067511297464593, -0.08927794634716622324, 6.802837160686558945E-17 ) ) ;
#9461=EDGE_CURVE ( 'NONE', #988, #534, #12869, .T. ) ;
#9468=DIRECTION ( 'NONE',  ( -6.158143864569485777E-17, -2.736152283717910599E-16, 1.000000000000000000 ) ) ;
#9470=DIRECTION ( 'NONE',  ( -0.6001121574638169642, 0.7999158696163758409, 1.927470528861191270E-16 ) ) ;
#9471=ADVANCED_FACE ( 'NONE', ( #1271 ), #6467, .T. ) ;
#9485=CARTESIAN_POINT ( 'NONE',  ( 50.92330601230504783, -13.90964864522661593, 2.499999999999996891 ) ) ;
#9486=ORIENTED_EDGE ( 'NONE', *, *, #4473, .F. ) ;
#9489=CARTESIAN_POINT ( 'NONE',  ( 34.99999999999958789, 1.104930248025249758E-13, -2.499999999999999112 ) ) ;
#9492=CARTESIAN_POINT ( 'NONE',  ( 26.09988479906369463, 19.17858047941126642, 2.500000000000004885 ) ) ;
#9515=DIRECTION ( 'NONE',  ( 0.000000000000000000, 0.000000000000000000, -1.000000000000000000 ) ) ;
#9518=EDGE_CURVE ( 'NONE', #4518, #6243, #8699, .T. ) ;
#9522=AXIS2_PLACEMENT_3D ( 'NONE', #11874, #5488, #7524 ) ;
#9523=EDGE_CURVE ( 'NONE', #4027, #7120, #8565, .T. ) ;
#9529=AXIS2_PLACEMENT_3D ( 'NONE', #3031, #12586, #2893 ) ;
#9554=EDGE_LOOP ( 'NONE', ( #5234, #999, #5396, #3596 ) ) ;
#9571=DIRECTION ( 'NONE',  ( -6.158143864569485777E-17, -2.736152283717910599E-16, 1.000000000000000000 ) ) ;
#9572=ORIENTED_EDGE ( 'NONE', *, *, #3182, .F. ) ;
#9590=DIRECTION ( 'NONE',  ( -6.158143864569485777E-17, -2.736152283717910599E-16, 1.000000000000000000 ) ) ;
#9593=AXIS2_PLACEMENT_3D ( 'NONE', #8810, #68, #3475 ) ;
#9597=EDGE_CURVE ( 'NONE', #3229, #4054, #9394, .T. ) ;
#9601=EDGE_CURVE ( 'NONE', #13485, #12269, #1777, .T. ) ;
#9613=CARTESIAN_POINT ( 'NONE',  ( 30.45476892764376231, 18.18971895053902443, 2.500000000000004885 ) ) ;
#9615=VECTOR ( 'NONE', #89, 1000.000000000000000 ) ;
#9632=CIRCLE ( 'NONE', #11210, 9.000000000008999024 ) ;
#9656=AXIS2_PLACEMENT_3D ( 'NONE', #8491, #11717, #735 ) ;
#9657=( LENGTH_UNIT ( ) NAMED_UNIT ( * ) SI_UNIT ( .MILLI., .METRE. ) );
#9666=VERTEX_POINT ( 'NONE', #11523 ) ;
#9667=EDGE_LOOP ( 'NONE', ( #13734, #9486, #13138, #9934 ) ) ;
#9669=DIRECTION ( 'NONE',  ( -6.158143864569485777E-17, -2.736152283717910599E-16, 1.000000000000000000 ) ) ;
#9673=EDGE_CURVE ( 'NONE', #3846, #4257, #11622, .T. ) ;
#9681=ORIENTED_EDGE ( 'NONE', *, *, #3809, .F. ) ;
#9685=DIRECTION ( 'NONE',  ( -6.158143864569485777E-17, -2.736152283717910599E-16, 1.000000000000000000 ) ) ;
#9688=DIRECTION ( 'NONE',  ( -6.158143864569485777E-17, -2.736152283717910599E-16, 1.000000000000000000 ) ) ;
#9690=DIRECTION ( 'NONE',  ( 0.7533101279583153120, -0.6576654553155629745, -1.387852799596036359E-16 ) ) ;
#9692=CARTESIAN_POINT ( 'NONE',  ( 155.9864723944028810, -111.6214737678657087, 2.500000000000000000 ) ) ;
#9693=EDGE_CURVE ( 'NONE', #4304, #12949, #12996, .T. ) ;
#9696=EDGE_CURVE ( 'NONE', #6030, #4257, #6697, .T. ) ;
#9697=CARTESIAN_POINT ( 'NONE',  ( 33.39358510189357787, -25.44935030951552690, -6.505213034913026604E-15 ) ) ;
#9703=CARTESIAN_POINT ( 'NONE',  ( 80.29381926039658879, -64.72749139719506672, 2.500000000000000000 ) ) ;
#9704=EDGE_LOOP ( 'NONE', ( #7677, #4648, #10813, #2286 ) ) ;
#9721=ORIENTED_EDGE ( 'NONE', *, *, #5335, .T. ) ;
#9724=ORIENTED_EDGE ( 'NONE', *, *, #1984, .F. ) ;
#9737=VECTOR ( 'NONE', #12817, 1000.000000000000000 ) ;
#9739=AXIS2_PLACEMENT_3D ( 'NONE', #8714, #469, #10880 ) ;
#9750=CIRCLE ( 'NONE', #13123, 25.50000000002549783 ) ;
#9757=CARTESIAN_POINT ( 'NONE',  ( 15.01254563088791372, -15.83514028494776404, -2.500000000000005329 ) ) ;
#9760=DIRECTION ( 'NONE',  ( -6.158143864569485777E-17, -2.736152283717910599E-16, 1.000000000000000000 ) ) ;
#9762=CARTESIAN_POINT ( 'NONE',  ( 23.90723890023449627, -15.11541108221136476, -2.500000000000003553 ) ) ;
#9766=CARTESIAN_POINT ( 'NONE',  ( 34.99999999999958789, 1.091249486606660213E-13, 2.500000000000000000 ) ) ;
#9767=ORIENTED_EDGE ( 'NONE', *, *, #6362, .F. ) ;
#9776=EDGE_CURVE ( 'NONE', #6151, #5594, #13230, .T. ) ;
#9778=CARTESIAN_POINT ( 'NONE',  ( 58.70736094381068426, -9.392073098158828515, 2.499999999999998668 ) ) ;
#9793=ORIENTED_EDGE ( 'NONE', *, *, #5840, .T. ) ;
#9794=DIRECTION ( 'NONE',  ( 6.158143864569485777E-17, 2.736152283717910599E-16, -1.000000000000000000 ) ) ;
#9810=CIRCLE ( 'NONE', #8257, 9.000000000008999024 ) ;
#9834=AXIS2_PLACEMENT_3D ( 'NONE', #4768, #6926, #13429 ) ;
#9854=CYLINDRICAL_SURFACE ( 'NONE', #13318, 25.50000000002549783 ) ;
#9861=VECTOR ( 'NONE', #7645, 1000.000000000000000 ) ;
#9863=VERTEX_POINT ( 'NONE', #10034 ) ;
#9885=DIRECTION ( 'NONE',  ( -6.158143864569485777E-17, -2.736152283717910599E-16, 1.000000000000000000 ) ) ;
#9897=PRODUCT ( 'Dual Pivoting Lever Wings (x2)', 'Dual Pivoting Lever Wings (x2)', '', ( #2351 ) ) ;
#9903=FACE_OUTER_BOUND ( 'NONE', #2127, .T. ) ;
#9929=VERTEX_POINT ( 'NONE', #7345 ) ;
#9934=ORIENTED_EDGE ( 'NONE', *, *, #5513, .T. ) ;
#9935=AXIS2_PLACEMENT_3D ( 'NONE', #8952, #13258, #3825 ) ;
#9953=AXIS2_PLACEMENT_3D ( 'NONE', #404, #7802, #12091 ) ;
#9956=CYLINDRICAL_SURFACE ( 'NONE', #4041, 18.74900000001875000 ) ;
#9969=ORIENTED_EDGE ( 'NONE', *, *, #5674, .F. ) ;
#9970=DIRECTION ( 'NONE',  ( -6.158143864569485777E-17, -2.736152283717910599E-16, 1.000000000000000000 ) ) ;
#9972=EDGE_CURVE ( 'NONE', #2032, #12858, #8278, .T. ) ;
#9975=FACE_OUTER_BOUND ( 'NONE', #10386, .T. ) ;
#9979=DIRECTION ( 'NONE',  ( -6.158143864569485777E-17, -2.736152283717910599E-16, 1.000000000000000000 ) ) ;
#9981=AXIS2_PLACEMENT_3D ( 'NONE', #609, #2702, #6977 ) ;
#9988=VECTOR ( 'NONE', #290, 1000.000000000000000 ) ;
#9989=DIRECTION ( 'NONE',  ( -6.158143864569485777E-17, -2.736152283717910599E-16, 1.000000000000000000 ) ) ;
#9992=ORIENTED_EDGE ( 'NONE', *, *, #4629, .T. ) ;
#9996=EDGE_CURVE ( 'NONE', #5217, #7956, #851, .T. ) ;
#9998=DIRECTION ( 'NONE',  ( -6.158143864569485777E-17, -2.736152283717910599E-16, 1.000000000000000000 ) ) ;
#10001=DIRECTION ( 'NONE',  ( -6.158143864569485777E-17, -2.736152283717910599E-16, 1.000000000000000000 ) ) ;
#10004=CARTESIAN_POINT ( 'NONE',  ( 34.99999999999958789, 1.091249486606660213E-13, 2.500000000000000000 ) ) ;
#10011=CARTESIAN_POINT ( 'NONE',  ( 55.20422767451771051, -6.230504303137470501, -2.499999999999999112 ) ) ;
#10017=ORIENTED_EDGE ( 'NONE', *, *, #7567, .T. ) ;
#10021=VERTEX_POINT ( 'NONE', #8415 ) ;
#10024=FACE_OUTER_BOUND ( 'NONE', #3648, .T. ) ;
#10025=CARTESIAN_POINT ( 'NONE',  ( 34.99999999999958789, 1.228057239789091624E-13, -47.50005079999998969 ) ) ;
#10034=CARTESIAN_POINT ( 'NONE',  ( 89.49979561504950709, -156.1132911148542917, -2.500000000000000000 ) ) ;
#10040=CIRCLE ( 'NONE', #7561, 9.000000000009000800 ) ;
#10041=DIRECTION ( 'NONE',  ( 6.158143864569485777E-17, 2.736152283717910599E-16, -1.000000000000000000 ) ) ;
#10046=CARTESIAN_POINT ( 'NONE',  ( 34.99999999999958789, 1.091249486606660213E-13, 2.500000000000000000 ) ) ;
#10056=ADVANCED_FACE ( 'NONE', ( #1374 ), #6635, .T. ) ;
#10058=CARTESIAN_POINT ( 'NONE',  ( 39.71817523509052705, -20.60992048131556942, -2.500000000000004441 ) ) ;
#10066=EDGE_CURVE ( 'NONE', #2729, #11081, #3617, .T. ) ;
#10070=DIRECTION ( 'NONE',  ( -6.158143864569485777E-17, -2.736152283717910599E-16, 1.000000000000000000 ) ) ;
#10071=ADVANCED_FACE ( 'NONE', ( #11049 ), #419, .F. ) ;
#10079=CARTESIAN_POINT ( 'NONE',  ( 17.19653809941365452, 5.878923826270381348, -2.499999999999999112 ) ) ;
#10084=CYLINDRICAL_SURFACE ( 'NONE', #8973, 9.000000000008999024 ) ;
#10086=AXIS2_PLACEMENT_3D ( 'NONE', #2394, #317, #4571 ) ;
#10092=DIRECTION ( 'NONE',  ( -0.9960067511297463483, 0.08927794634716618161, -4.818676322152979407E-17 ) ) ;
#10094=CIRCLE ( 'NONE', #2029, 9.000000000009000800 ) ;
#10102=VECTOR ( 'NONE', #10001, 1000.000000000000000 ) ;
#10104=ORIENTED_EDGE ( 'NONE', *, *, #90, .T. ) ;
#10109=ORIENTED_EDGE ( 'NONE', *, *, #8641, .F. ) ;
#10113=EDGE_LOOP ( 'NONE', ( #3245, #1455, #682, #439 ) ) ;
#10121=FACE_OUTER_BOUND ( 'NONE', #10113, .T. ) ;
#10124=ORIENTED_EDGE ( 'NONE', *, *, #9696, .F. ) ;
#10130=EDGE_CURVE ( 'NONE', #1977, #4304, #2325, .T. ) ;
#10149=ORIENTED_EDGE ( 'NONE', *, *, #9972, .F. ) ;
#10158=LINE ( 'NONE', #1736, #10536 ) ;
#10162=DIRECTION ( 'NONE',  ( 0.9960067511297463483, -0.08927794634716620936, 4.626175998653454121E-17 ) ) ;
#10167=ORIENTED_EDGE ( 'NONE', *, *, #1652, .F. ) ;
#10171=DIRECTION ( 'NONE',  ( -6.158143864569485777E-17, -2.736152283717910599E-16, 1.000000000000000000 ) ) ;
#10176=AXIS2_PLACEMENT_3D ( 'NONE', #12033, #4520, #10973 ) ;
#10195=ORIENTED_EDGE ( 'NONE', *, *, #13612, .F. ) ;
#10197=CARTESIAN_POINT ( 'NONE',  ( 52.27091746333575628, 18.76074118940758240, -2.499999999999992895 ) ) ;
#10198=CARTESIAN_POINT ( 'NONE',  ( 57.84299132690245671, 11.33347904398043049, -2.499999999999994671 ) ) ;
#10199=CARTESIAN_POINT ( 'NONE',  ( 22.31663499682298735, 16.91633092580596198, 2.500000000000003997 ) ) ;
#10206=DIRECTION ( 'NONE',  ( 1.000000000000000000, 0.000000000000000000, 0.000000000000000000 ) ) ;
#10212=AXIS2_PLACEMENT_3D ( 'NONE', #7025, #8926, #6747 ) ;
#10220=ORIENTED_EDGE ( 'NONE', *, *, #10567, .F. ) ;
#10230=ORIENTED_EDGE ( 'NONE', *, *, #7122, .T. ) ;
#10231=ORIENTED_EDGE ( 'NONE', *, *, #13499, .F. ) ;
#10242=ORIENTED_EDGE ( 'NONE', *, *, #2844, .T. ) ;
#10282=ORIENTED_EDGE ( 'NONE', *, *, #8834, .F. ) ;
#10288=CLOSED_SHELL ( 'NONE', ( #11679, #4342, #13060, #7958, #7491, #6510, #10071, #9110, #9418, #11508, #1992, #12170, #2142, #2156, #4294, #13371, #6021, #10309, #1482, #12614, #2865, #12529, #646, #12801, #11411, #4886, #6203, #13353, #10056, #3090, #12187, #6451, #1585, #9471, #11413, #6057, #5240, #6967, #2930, #8528, #11238, #6769, #9357, #9216, #7743, #11174, #7043, #197, #8659, #88, #3959, #1384, #4905, #4669, #6420, #13777, #10731, #12090, #12080, #3961, #2377, #4025, #11033, #6370, #11585, #7308 ) ) ;
#10289=EDGE_CURVE ( 'NONE', #13160, #3229, #3763, .T. ) ;
#10291=CYLINDRICAL_SURFACE ( 'NONE', #8211, 25.50000000002549783 ) ;
#10293=CARTESIAN_POINT ( 'NONE',  ( 51.25836974494252019, 19.64472991003004054, -2.499999999999992450 ) ) ;
#10305=VECTOR ( 'NONE', #2295, 1000.000000000000000 ) ;
#10309=ADVANCED_FACE ( 'NONE', ( #3973 ), #7394, .T. ) ;
#10312=LINE ( 'NONE', #4185, #7340 ) ;
#10316=VECTOR ( 'NONE', #1569, 1000.000000000000114 ) ;
#10327=CARTESIAN_POINT ( 'NONE',  ( 31.01425004688410070, -18.32044754671509423, 2.499999999999994671 ) ) ;
#10330=LINE ( 'NONE', #731, #7974 ) ;
#10331=ORIENTED_EDGE ( 'NONE', *, *, #4816, .F. ) ;
#10333=ORIENTED_EDGE ( 'NONE', *, *, #456, .F. ) ;
#10340=ORIENTED_EDGE ( 'NONE', *, *, #6303, .F. ) ;
#10349=CARTESIAN_POINT ( 'NONE',  ( 10.29982004912477578, -6.336490384724132952, 2.499999999999996447 ) ) ;
#10370=PLANE ( 'NONE',  #76 ) ;
#10372=DIRECTION ( 'NONE',  ( 0.5753203450992270263, 0.8179281756455796248, 2.409338161076488717E-16 ) ) ;
#10375=VECTOR ( 'NONE', #5907, 1000.000000000000000 ) ;
#10381=ORIENTED_EDGE ( 'NONE', *, *, #2309, .T. ) ;
#10386=EDGE_LOOP ( 'NONE', ( #13634, #12654, #6242, #6232 ) ) ;
#10388=ORIENTED_EDGE ( 'NONE', *, *, #3318, .F. ) ;
#10391=CYLINDRICAL_SURFACE ( 'NONE', #3417, 9.000000000008999024 ) ;
#10395=DIRECTION ( 'NONE',  ( -0.9960067511297463483, 0.08927794634716618161, -4.818676322152979407E-17 ) ) ;
#10397=DIRECTION ( 'NONE',  ( -6.158143864569485777E-17, -2.736152283717910599E-16, 1.000000000000000000 ) ) ;
#10412=CARTESIAN_POINT ( 'NONE',  ( 34.99999999999958789, 1.104930248025249758E-13, -2.499999999999999112 ) ) ;
#10415=ORIENTED_EDGE ( 'NONE', *, *, #5233, .T. ) ;
#10419=EDGE_CURVE ( 'NONE', #425, #1659, #2571, .T. ) ;
#10420=ORIENTED_EDGE ( 'NONE', *, *, #12452, .T. ) ;
#10425=DIRECTION ( 'NONE',  ( -6.158143864569485777E-17, -2.736152283717910599E-16, 1.000000000000000000 ) ) ;
#10450=AXIS2_PLACEMENT_3D ( 'NONE', #1737, #7265, #4043 ) ;
#10453=VERTEX_POINT ( 'NONE', #7326 ) ;
#10457=DIRECTION ( 'NONE',  ( -0.9462100554738961389, -0.3235529800822217195, -1.387852799596036113E-16 ) ) ;
#10465=DIRECTION ( 'NONE',  ( -0.9960067511297463483, 0.08927794634716618161, -4.818676322152979407E-17 ) ) ;
#10479=DIRECTION ( 'NONE',  ( -6.158143864569485777E-17, -2.736152283717910599E-16, 1.000000000000000000 ) ) ;
#10491=DIRECTION ( 'NONE',  ( 0.4226182617407009401, -0.9063077870366491595, -0.000000000000000000 ) ) ;
#10503=CARTESIAN_POINT ( 'NONE',  ( 35.66405164569891184, -18.73723662690267133, -2.500000000000004441 ) ) ;
#10507=CIRCLE ( 'NONE', #4030, 18.74900000001875355 ) ;
#10509=ORIENTED_EDGE ( 'NONE', *, *, #13761, .F. ) ;
#10511=CIRCLE ( 'NONE', #1037, 25.50000000002549783 ) ;
#10512=EDGE_LOOP ( 'NONE', ( #8375, #9260, #7294, #11020 ) ) ;
#10520=CARTESIAN_POINT ( 'NONE',  ( 62.16766351966359849, -73.17985663200910551, 2.500000000000000000 ) ) ;
#10522=AXIS2_PLACEMENT_3D ( 'NONE', #926, #3941, #5064 ) ;
#10528=AXIS2_PLACEMENT_3D ( 'NONE', #13144, #2380, #2177 ) ;
#10530=VERTEX_POINT ( 'NONE', #7667 ) ;
#10534=CARTESIAN_POINT ( 'NONE',  ( 50.89489709276795537, 9.943703908052052398, -2.499999999999994671 ) ) ;
#10536=VECTOR ( 'NONE', #9167, 1000.000000000000000 ) ;
#10538=CYLINDRICAL_SURFACE ( 'NONE', #1106, 9.000000000008999024 ) ;
#10545=CARTESIAN_POINT ( 'NONE',  ( 31.01425004688410070, -18.32044754671509423, -2.500000000000004441 ) ) ;
#10549=DIRECTION ( 'NONE',  ( -6.158143864569485777E-17, -2.736152283717910599E-16, 1.000000000000000000 ) ) ;
#10554=EDGE_CURVE ( 'NONE', #11257, #5704, #7595, .T. ) ;
#10561=AXIS2_PLACEMENT_3D ( 'NONE', #1336, #9760, #2539 ) ;
#10567=EDGE_CURVE ( 'NONE', #13160, #6892, #339, .T. ) ;
#10577=ORIENTED_EDGE ( 'NONE', *, *, #11330, .F. ) ;
#10592=VECTOR ( 'NONE', #11613, 1000.000000000000000 ) ;
#10600=CIRCLE ( 'NONE', #13562, 9.000000000008999024 ) ;
#10604=DIRECTION ( 'NONE',  ( 0.9960067511297463483, -0.08927794634716620936, 4.818676322152979407E-17 ) ) ;
#10605=CARTESIAN_POINT ( 'NONE',  ( 76.84607712649204814, -99.92541302764922762, -2.500000000000000000 ) ) ;
#10629=AXIS2_PLACEMENT_3D ( 'NONE', #11322, #11383, #12244 ) ;
#10635=AXIS2_PLACEMENT_3D ( 'NONE', #10058, #5927, #13241 ) ;
#10644=ORIENTED_EDGE ( 'NONE', *, *, #5335, .F. ) ;
#10650=ORIENTED_EDGE ( 'NONE', *, *, #3780, .F. ) ;
#10653=CIRCLE ( 'NONE', #5504, 18.74900000001875000 ) ;
#10658=DIRECTION ( 'NONE',  ( -6.158143864569485777E-17, -2.736152283717910599E-16, 1.000000000000000000 ) ) ;
#10659=ORIENTED_EDGE ( 'NONE', *, *, #9461, .T. ) ;
#10660=EDGE_CURVE ( 'NONE', #12400, #11019, #3385, .T. ) ;
#10666=ORIENTED_EDGE ( 'NONE', *, *, #3093, .F. ) ;
#10688=DIRECTION ( 'NONE',  ( 0.9960067511297464593, -0.08927794634716622324, 3.401418580343279473E-17 ) ) ;
#10690=VECTOR ( 'NONE', #6304, 1000.000000000000000 ) ;
#10693=EDGE_CURVE ( 'NONE', #4720, #2860, #12215, .T. ) ;
#10698=CARTESIAN_POINT ( 'NONE',  ( 53.02537423504344360, -5.158573900538657497, -2.499999999999999112 ) ) ;
#10703=ORIENTED_EDGE ( 'NONE', *, *, #13052, .T. ) ;
#10705=EDGE_CURVE ( 'NONE', #6547, #5305, #1574, .T. ) ;
#10711=LINE ( 'NONE', #12048, #13274 ) ;
#10722=ORIENTED_EDGE ( 'NONE', *, *, #6851, .T. ) ;
#10726=CARTESIAN_POINT ( 'NONE',  ( 34.99999999999958789, 1.104930248025249758E-13, -2.499999999999999112 ) ) ;
#10731=ADVANCED_FACE ( 'NONE', ( #9903 ), #13079, .T. ) ;
#10732=CARTESIAN_POINT ( 'NONE',  ( 16.85679715600144135, -10.85606698379831947, -2.500000000000003553 ) ) ;
#10733=AXIS2_PLACEMENT_3D ( 'NONE', #13406, #4740, #10206 ) ;
#10741=DIRECTION ( 'NONE',  ( -6.158143864569485777E-17, -2.736152283717910599E-16, 1.000000000000000000 ) ) ;
#10744=LINE ( 'NONE', #1221, #2012 ) ;
#10746=ORIENTED_EDGE ( 'NONE', *, *, #3677, .F. ) ;
#10750=CYLINDRICAL_SURFACE ( 'NONE', #13809, 25.50000000002549783 ) ;
#10752=DIRECTION ( 'NONE',  ( -6.158143864569485777E-17, -2.736152283717910599E-16, 1.000000000000000000 ) ) ;
#10756=FACE_OUTER_BOUND ( 'NONE', #7067, .T. ) ;
#10760=VECTOR ( 'NONE', #11316, 1000.000000000000000 ) ;
#10766=CIRCLE ( 'NONE', #10561, 18.74900000001875711 ) ;
#10768=DIRECTION ( 'NONE',  ( -0.2228746399763467390, 0.9748471135800802490, 2.409338161076489210E-16 ) ) ;
#10775=ORIENTED_EDGE ( 'NONE', *, *, #8816, .F. ) ;
#10801=CARTESIAN_POINT ( 'NONE',  ( 34.99999999999958789, 1.104930248025249758E-13, -2.499999999999999112 ) ) ;
#10809=CARTESIAN_POINT ( 'NONE',  ( 22.00707094244967621, -21.94159963418280412, -2.500000000000005329 ) ) ;
#10813=ORIENTED_EDGE ( 'NONE', *, *, #10885, .F. ) ;
#10816=AXIS2_PLACEMENT_3D ( 'NONE', #6814, #11011, #5836 ) ;
#10821=AXIS2_PLACEMENT_3D ( 'NONE', #344, #4603, #13192 ) ;
#10822=FACE_OUTER_BOUND ( 'NONE', #13358, .T. ) ;
#10824=EDGE_CURVE ( 'NONE', #4918, #9172, #5263, .T. ) ;
#10828=SURFACE_STYLE_USAGE ( .BOTH. , #11821 ) ;
#10833=DIRECTION ( 'NONE',  ( -6.158143864569485777E-17, -2.736152283717910599E-16, 1.000000000000000000 ) ) ;
#10844=ORIENTED_EDGE ( 'NONE', *, *, #12901, .T. ) ;
#10849=DIRECTION ( 'NONE',  ( -6.158143864569485777E-17, -2.736152283717910599E-16, 1.000000000000000000 ) ) ;
#10860=EDGE_LOOP ( 'NONE', ( #13321, #2850, #6342, #2764, #10381, #7552, #314, #7050, #12257, #11130, #11230, #3409, #5976, #2365, #6061, #11848, #4579, #7818, #12035, #11374, #10415, #3831, #242, #5453, #11975, #11154, #1842, #7594, #6751, #11992, #11061, #12491, #3886, #8806, #12280, #11333, #3144, #2782, #294, #5974, #13319, #12399, #5353, #1074, #4685, #7150, #1860, #9213, #10844, #10388, #9158, #12655, #5739, #1494, #3874, #13815, #8908, #4259, #4840, #5532, #2033, #13690 ) ) ;
#10861=CARTESIAN_POINT ( 'NONE',  ( 34.99999999999958789, 1.063887963769481123E-13, 12.50000000000000000 ) ) ;
#10867=DIRECTION ( 'NONE',  ( -6.158143864569485777E-17, -2.736152283717910599E-16, 1.000000000000000000 ) ) ;
#10879=ORIENTED_EDGE ( 'NONE', *, *, #7977, .F. ) ;
#10880=DIRECTION ( 'NONE',  ( -0.7328050451781167318, -0.6804386568688601811, -2.409338161076489703E-16 ) ) ;
#10885=EDGE_CURVE ( 'NONE', #2631, #5397, #824, .T. ) ;
#10893=ORIENTED_EDGE ( 'NONE', *, *, #1966, .T. ) ;
#10894=EDGE_CURVE ( 'NONE', #9929, #5202, #1023, .T. ) ;
#10895=ORIENTED_EDGE ( 'NONE', *, *, #4175, .F. ) ;
#10903=DIRECTION ( 'NONE',  ( -6.158143864569485777E-17, -2.736152283717910599E-16, 1.000000000000000000 ) ) ;
#10911=AXIS2_PLACEMENT_3D ( 'NONE', #530, #12151, #5767 ) ;
#10913=CARTESIAN_POINT ( 'NONE',  ( 18.44105126153190710, 8.793532718851093222, 2.500000000000001332 ) ) ;
#10916=LINE ( 'NONE', #13211, #9988 ) ;
#10917=DIRECTION ( 'NONE',  ( -6.158143864569485777E-17, -2.736152283717910599E-16, 1.000000000000000000 ) ) ;
#10919=DIRECTION ( 'NONE',  ( -0.4226182617407014397, 0.9063077870366489375, 0.000000000000000000 ) ) ;
#10925=DIRECTION ( 'NONE',  ( 0.9960067511297464593, -0.08927794634716622324, 3.401418580343279473E-17 ) ) ;
#10927=DIRECTION ( 'NONE',  ( 1.000000000000000000, 0.000000000000000000, 0.000000000000000000 ) ) ;
#10929=ORIENTED_EDGE ( 'NONE', *, *, #704, .T. ) ;
#10931=DIRECTION ( 'NONE',  ( 0.000000000000000000, 0.000000000000000000, 1.000000000000000000 ) ) ;
#10938=AXIS2_PLACEMENT_3D ( 'NONE', #8798, #12177, #7895 ) ;
#10939=DIRECTION ( 'NONE',  ( 0.9556796851544553384, -0.2944084567112177364, -2.313087999326726136E-17 ) ) ;
#10944=CARTESIAN_POINT ( 'NONE',  ( 16.29599561779310335, 1.298160649189404880, -2.500000000000000000 ) ) ;
#10948=DIRECTION ( 'NONE',  ( -6.158143864569485777E-17, -2.736152283717910599E-16, 1.000000000000000000 ) ) ;
#10962=DIRECTION ( 'NONE',  ( 6.158143864569485777E-17, 2.736152283717910599E-16, -1.000000000000000000 ) ) ;
#10963=EDGE_CURVE ( 'NONE', #2483, #4263, #6152, .T. ) ;
#10966=ORIENTED_EDGE ( 'NONE', *, *, #3842, .T. ) ;
#10969=ORIENTED_EDGE ( 'NONE', *, *, #1118, .T. ) ;
#10973=DIRECTION ( 'NONE',  ( 0.9960067511297463483, -0.08927794634716618161, 4.818676322152979407E-17 ) ) ;
#10977=FACE_OUTER_BOUND ( 'NONE', #3991, .T. ) ;
#10987=EDGE_LOOP ( 'NONE', ( #2360, #10644, #4593, #838 ) ) ;
#11004=CIRCLE ( 'NONE', #1835, 18.74900000001875355 ) ;
#11007=CARTESIAN_POINT ( 'NONE',  ( 22.00707094244967621, -21.94159963418280057, 2.499999999999992895 ) ) ;
#11009=CARTESIAN_POINT ( 'NONE',  ( 76.84607712649204814, -99.92541302764922762, 2.500000000000000000 ) ) ;
#11011=DIRECTION ( 'NONE',  ( -6.158143864569485777E-17, -2.736152283717910599E-16, 1.000000000000000000 ) ) ;
#11014=CARTESIAN_POINT ( 'NONE',  ( 23.44929957547844879, 14.76842309468663750, -2.499999999999996447 ) ) ;
#11018=DIRECTION ( 'NONE',  ( -6.158143864569485777E-17, -2.736152283717910599E-16, 1.000000000000000000 ) ) ;
#11019=VERTEX_POINT ( 'NONE', #319 ) ;
#11020=ORIENTED_EDGE ( 'NONE', *, *, #723, .T. ) ;
#11022=DIRECTION ( 'NONE',  ( 0.7533101279583153120, -0.6576654553155628635, -1.445602896645893822E-16 ) ) ;
#11033=ADVANCED_FACE ( 'NONE', ( #1224 ), #6614, .T. ) ;
#11041=VECTOR ( 'NONE', #929, 1000.000000000000000 ) ;
#11049=FACE_OUTER_BOUND ( 'NONE', #6397, .T. ) ;
#11052=EDGE_CURVE ( 'NONE', #3832, #182, #8401, .T. ) ;
#11061=ORIENTED_EDGE ( 'NONE', *, *, #1816, .T. ) ;
#11066=ORIENTED_EDGE ( 'NONE', *, *, #8493, .F. ) ;
#11067=EDGE_CURVE ( 'NONE', #7956, #2525, #11320, .T. ) ;
#11072=AXIS2_PLACEMENT_3D ( 'NONE', #12598, #7112, #6141 ) ;
#11077=LINE ( 'NONE', #1469, #9259 ) ;
#11079=VERTEX_POINT ( 'NONE', #10809 ) ;
#11081=VERTEX_POINT ( 'NONE', #12083 ) ;
#11091=AXIS2_PLACEMENT_3D ( 'NONE', #2698, #11380, #6974 ) ;
#11106=DIRECTION ( 'NONE',  ( 0.9960067511297464593, -0.08927794634716622324, 6.802837160686558945E-17 ) ) ;
#11130=ORIENTED_EDGE ( 'NONE', *, *, #11067, .T. ) ;
#11142=ORIENTED_EDGE ( 'NONE', *, *, #1652, .T. ) ;
#11145=PRODUCT_DEFINITION ( 'UNKNOWN', '', #13137, #2510 ) ;
#11147=VERTEX_POINT ( 'NONE', #10198 ) ;
#11154=ORIENTED_EDGE ( 'NONE', *, *, #1279, .F. ) ;
#11156=EDGE_LOOP ( 'NONE', ( #1344, #12029, #13622, #10969 ) ) ;
#11174=ADVANCED_FACE ( 'NONE', ( #4867 ), #2553, .T. ) ;
#11178=AXIS2_PLACEMENT_3D ( 'NONE', #3370, #7652, #11929 ) ;
#11210=AXIS2_PLACEMENT_3D ( 'NONE', #1163, #10948, #3450 ) ;
#11213=ORIENTED_EDGE ( 'NONE', *, *, #1564, .T. ) ;
#11218=ORIENTED_EDGE ( 'NONE', *, *, #1279, .T. ) ;
#11230=ORIENTED_EDGE ( 'NONE', *, *, #3163, .T. ) ;
#11238=ADVANCED_FACE ( 'NONE', ( #11255 ), #12383, .T. ) ;
#11239=DIRECTION ( 'NONE',  ( -0.9063077870366490485, -0.4226182617407014952, 0.000000000000000000 ) ) ;
#11251=VERTEX_POINT ( 'NONE', #2833 ) ;
#11254=LINE ( 'NONE', #5925, #10760 ) ;
#11255=FACE_OUTER_BOUND ( 'NONE', #2545, .T. ) ;
#11257=VERTEX_POINT ( 'NONE', #4803 ) ;
#11261=EDGE_CURVE ( 'NONE', #13136, #988, #6846, .T. ) ;
#11263=DIRECTION ( 'NONE',  ( -6.158143864569485777E-17, -2.736152283717910599E-16, 1.000000000000000000 ) ) ;
#11265=FACE_BOUND ( 'NONE', #4078, .T. ) ;
#11276=DIRECTION ( 'NONE',  ( -6.158143864569485777E-17, -2.736152283717910599E-16, 1.000000000000000000 ) ) ;
#11281=ORIENTED_EDGE ( 'NONE', *, *, #7205, .F. ) ;
#11282=AXIS2_PLACEMENT_3D ( 'NONE', #4070, #6250, #12646 ) ;
#11292=ORIENTED_EDGE ( 'NONE', *, *, #6984, .T. ) ;
#11306=ORIENTED_EDGE ( 'NONE', *, *, #4228, .T. ) ;
#11316=DIRECTION ( 'NONE',  ( -6.158143864569485777E-17, -2.736152283717910599E-16, 1.000000000000000000 ) ) ;
#11318=LINE ( 'NONE', #12443, #10316 ) ;
#11320=CIRCLE ( 'NONE', #9302, 9.000000000009000800 ) ;
#11322=CARTESIAN_POINT ( 'NONE',  ( 30.29366116764611760, 20.61262658154624816, -2.499999999999993783 ) ) ;
#11330=EDGE_CURVE ( 'NONE', #12858, #3661, #11549, .T. ) ;
#11333=ORIENTED_EDGE ( 'NONE', *, *, #9363, .T. ) ;
#11353=CIRCLE ( 'NONE', #8663, 9.000000000009000800 ) ;
#11370=AXIS2_PLACEMENT_3D ( 'NONE', #7753, #9590, #1248 ) ;
#11374=ORIENTED_EDGE ( 'NONE', *, *, #4890, .T. ) ;
#11376=VERTEX_POINT ( 'NONE', #389 ) ;
#11380=DIRECTION ( 'NONE',  ( -6.158143864569485777E-17, -2.736152283717910599E-16, 1.000000000000000000 ) ) ;
#11383=DIRECTION ( 'NONE',  ( -6.158143864569485777E-17, -2.736152283717910599E-16, 1.000000000000000000 ) ) ;
#11387=EDGE_CURVE ( 'NONE', #8296, #11257, #6613, .T. ) ;
#11391=AXIS2_PLACEMENT_3D ( 'NONE', #4991, #13584, #12224 ) ;
#11411=ADVANCED_FACE ( 'NONE', ( #9067 ), #3800, .T. ) ;
#11413=ADVANCED_FACE ( 'NONE', ( #8088 ), #2754, .T. ) ;
#11421=VECTOR ( 'NONE', #378, 1000.000000000000000 ) ;
#11429=AXIS2_PLACEMENT_3D ( 'NONE', #4973, #6105, #10372 ) ;
#11431=ORIENTED_EDGE ( 'NONE', *, *, #3852, .F. ) ;
#11432=DIRECTION ( 'NONE',  ( 0.9960067511297463483, -0.08927794634716618161, 4.818676322152979407E-17 ) ) ;
#11448=DIRECTION ( 'NONE',  ( -6.158143864569485777E-17, -2.736152283717910599E-16, 1.000000000000000000 ) ) ;
#11452=VERTEX_POINT ( 'NONE', #928 ) ;
#11454=AXIS2_PLACEMENT_3D ( 'NONE', #11794, #5078, #13872 ) ;
#11455=AXIS2_PLACEMENT_3D ( 'NONE', #5416, #7878, #13012 ) ;
#11470=VERTEX_POINT ( 'NONE', #3088 ) ;
#11490=CIRCLE ( 'NONE', #11918, 18.74900000001875000 ) ;
#11492=CARTESIAN_POINT ( 'NONE',  ( 35.65577094119244350, -20.24578327824959345, 2.499999999999994671 ) ) ;
#11498=CARTESIAN_POINT ( 'NONE',  ( 56.05919550416194141, -1.881564379087037553, -2.499999999999998224 ) ) ;
#11500=VERTEX_POINT ( 'NONE', #1700 ) ;
#11505=ORIENTED_EDGE ( 'NONE', *, *, #6515, .F. ) ;
#11508=ADVANCED_FACE ( 'NONE', ( #7299 ), #3868, .T. ) ;
#11509=FACE_OUTER_BOUND ( 'NONE', #358, .T. ) ;
#11515=CARTESIAN_POINT ( 'NONE',  ( 34.99999999999958789, 1.091249486606660213E-13, 2.500000000000000000 ) ) ;
#11517=DIRECTION ( 'NONE',  ( -6.158143864569485777E-17, -2.736152283717910599E-16, 1.000000000000000000 ) ) ;
#11523=CARTESIAN_POINT ( 'NONE',  ( 33.39358510189357787, -25.44935030951552690, 2.499999999999992895 ) ) ;
#11540=ORIENTED_EDGE ( 'NONE', *, *, #3677, .T. ) ;
#11544=DIRECTION ( 'NONE',  ( 0.9960067511297464593, -0.08927794634716622324, 3.401418580343279473E-17 ) ) ;
#11549=CIRCLE ( 'NONE', #7284, 18.74900000001875355 ) ;
#11551=FACE_OUTER_BOUND ( 'NONE', #13118, .T. ) ;
#11556=AXIS2_PLACEMENT_3D ( 'NONE', #1906, #791, #4993 ) ;
#11560=DIRECTION ( 'NONE',  ( -6.158143864569485777E-17, -2.736152283717910599E-16, 1.000000000000000000 ) ) ;
#11562=DIRECTION ( 'NONE',  ( -6.158143864569485777E-17, -2.736152283717910599E-16, 1.000000000000000000 ) ) ;
#11563=DIRECTION ( 'NONE',  ( 0.9960067511297463483, -0.08927794634716618161, 4.818676322152979407E-17 ) ) ;
#11568=VERTEX_POINT ( 'NONE', #10327 ) ;
#11569=VERTEX_POINT ( 'NONE', #8425 ) ;
#11572=VERTEX_POINT ( 'NONE', #9412 ) ;
#11575=CARTESIAN_POINT ( 'NONE',  ( 50.92330601230504783, -13.90964864522661415, -2.500000000000001776 ) ) ;
#11580=CARTESIAN_POINT ( 'NONE',  ( 52.85884796071297131, 5.708463060827149604, -2.499999999999996447 ) ) ;
#11581=EDGE_CURVE ( 'NONE', #5397, #9929, #13833, .T. ) ;
#11583=EDGE_CURVE ( 'NONE', #11832, #11754, #10653, .T. ) ;
#11585=ADVANCED_FACE ( 'NONE', ( #9206 ), #12713, .T. ) ;
#11601=LINE ( 'NONE', #10545, #8548 ) ;
#11607=ORIENTED_EDGE ( 'NONE', *, *, #1340, .T. ) ;
#11608=FACE_OUTER_BOUND ( 'NONE', #12047, .T. ) ;
#11613=DIRECTION ( 'NONE',  ( 0.000000000000000000, 0.000000000000000000, -1.000000000000000000 ) ) ;
#11620=DIRECTION ( 'NONE',  ( -0.9960067511297463483, 0.08927794634716618161, -4.818676322152979407E-17 ) ) ;
#11622=CIRCLE ( 'NONE', #8703, 9.000000000008999024 ) ;
#11628=EDGE_LOOP ( 'NONE', ( #12282, #13504, #85, #8932 ) ) ;
#11649=CIRCLE ( 'NONE', #3566, 80.00000000000001421 ) ;
#11658=DIRECTION ( 'NONE',  ( -6.158143864569485777E-17, -2.736152283717910599E-16, 1.000000000000000000 ) ) ;
#11667=DIRECTION ( 'NONE',  ( -6.158143864569485777E-17, -2.736152283717910599E-16, 1.000000000000000000 ) ) ;
#11675=DIRECTION ( 'NONE',  ( 0.9960067511297464593, -0.08927794634716622324, 6.802837160686558945E-17 ) ) ;
#11679=ADVANCED_FACE ( 'NONE', ( #13129 ), #9050, .F. ) ;
#11680=VECTOR ( 'NONE', #6432, 1000.000000000000000 ) ;
#11697=ORIENTED_EDGE ( 'NONE', *, *, #9601, .F. ) ;
#11701=VECTOR ( 'NONE', #10903, 1000.000000000000000 ) ;
#11703=CIRCLE ( 'NONE', #12398, 2.500000000000000444 ) ;
#11704=CARTESIAN_POINT ( 'NONE',  ( 34.99999999999958789, 1.091249486606660213E-13, 2.500000000000000000 ) ) ;
#11711=CARTESIAN_POINT ( 'NONE',  ( 14.00979921278056040, -2.538005261501627086, -2.500000000000000888 ) ) ;
#11717=DIRECTION ( 'NONE',  ( 0.000000000000000000, 0.000000000000000000, 1.000000000000000000 ) ) ;
#11754=VERTEX_POINT ( 'NONE', #5898 ) ;
#11757=EDGE_CURVE ( 'NONE', #3278, #9863, #10916, .T. ) ;
#11758=( NAMED_UNIT ( * ) PLANE_ANGLE_UNIT ( ) SI_UNIT ( $, .RADIAN. ) );
#11763=CIRCLE ( 'NONE', #3708, 9.000000000009002576 ) ;
#11775=EDGE_CURVE ( 'NONE', #9058, #7693, #4845, .T. ) ;
#11780=DIRECTION ( 'NONE',  ( -6.158143864569485777E-17, -2.736152283717910599E-16, 1.000000000000000000 ) ) ;
#11787=DIRECTION ( 'NONE',  ( -0.9960067511297463483, 0.08927794634716618161, -4.818676322152979407E-17 ) ) ;
#11794=CARTESIAN_POINT ( 'NONE',  ( 34.99999999999958789, 1.091249486606660213E-13, 2.500000000000000000 ) ) ;
#11804=ORIENTED_EDGE ( 'NONE', *, *, #6600, .F. ) ;
#11807=CYLINDRICAL_SURFACE ( 'NONE', #3021, 9.000000000008999024 ) ;
#11808=CARTESIAN_POINT ( 'NONE',  ( 34.99999999999958789, 1.063887963769481123E-13, 12.50000000000000000 ) ) ;
#11817=ORIENTED_EDGE ( 'NONE', *, *, #5450, .F. ) ;
#11821=SURFACE_SIDE_STYLE ('',( #1177 ) ) ;
#11829=VECTOR ( 'NONE', #13893, 1000.000000000000000 ) ;
#11832=VERTEX_POINT ( 'NONE', #1819 ) ;
#11839=VECTOR ( 'NONE', #10425, 1000.000000000000000 ) ;
#11843=EDGE_CURVE ( 'NONE', #1753, #9666, #7740, .T. ) ;
#11848=ORIENTED_EDGE ( 'NONE', *, *, #11387, .T. ) ;
#11850=VERTEX_POINT ( 'NONE', #1100 ) ;
#11860=CARTESIAN_POINT ( 'NONE',  ( 22.84091969677297485, -17.29701610032388359, 2.499999999999994227 ) ) ;
#11871=COLOUR_RGB ( '', 0.31764706, 0.68627451, 0.89019608) ;
#11874=CARTESIAN_POINT ( 'NONE',  ( 55.00383357371546822, 6.846651893462920135, -2.499999999999995559 ) ) ;
#11887=CARTESIAN_POINT ( 'NONE',  ( 50.48962708925064646, 14.39101985375337556, -2.499999999999993783 ) ) ;
#11888=AXIS2_PLACEMENT_3D ( 'NONE', #3514, #12305, #8939 ) ;
#11899=DIRECTION ( 'NONE',  ( -6.158143864569485777E-17, -2.736152283717910599E-16, 1.000000000000000000 ) ) ;
#11906=ORIENTED_EDGE ( 'NONE', *, *, #796, .T. ) ;
#11908=DIRECTION ( 'NONE',  ( 0.9960067511297463483, -0.08927794634716618161, 4.818676322152979407E-17 ) ) ;
#11911=DIRECTION ( 'NONE',  ( -6.158143864569485777E-17, -2.736152283717910599E-16, 1.000000000000000000 ) ) ;
#11918=AXIS2_PLACEMENT_3D ( 'NONE', #8526, #189, #5564 ) ;
#11929=DIRECTION ( 'NONE',  ( 0.9960067511297463483, -0.08927794634716620936, 4.626175998653454121E-17 ) ) ;
#11930=FACE_OUTER_BOUND ( 'NONE', #5670, .T. ) ;
#11933=DIRECTION ( 'NONE',  ( 6.158143864569485777E-17, 2.736152283717910599E-16, -1.000000000000000000 ) ) ;
#11949=CARTESIAN_POINT ( 'NONE',  ( 21.12690199240172007, 12.61198448588842247, 2.500000000000002665 ) ) ;
#11965=AXIS2_PLACEMENT_3D ( 'NONE', #11808, #1940, #2132 ) ;
#11973=EDGE_LOOP ( 'NONE', ( #2506, #9767, #7124, #1290 ) ) ;
#11975=ORIENTED_EDGE ( 'NONE', *, *, #12447, .T. ) ;
#11979=CARTESIAN_POINT ( 'NONE',  ( 55.16425081158429577, -10.83695794929873912, -2.500000000000000000 ) ) ;
#11984=CARTESIAN_POINT ( 'NONE',  ( 34.99999999999958789, 1.091249486606660213E-13, 2.500000000000000000 ) ) ;
#11986=ORIENTED_EDGE ( 'NONE', *, *, #12735, .F. ) ;
#11987=DIRECTION ( 'NONE',  ( 0.9960067511297464593, -0.08927794634716622324, 3.401418580343279473E-17 ) ) ;
#11991=DIRECTION ( 'NONE',  ( 6.158143864569485777E-17, 2.736152283717910599E-16, -1.000000000000000000 ) ) ;
#11992=ORIENTED_EDGE ( 'NONE', *, *, #4228, .F. ) ;
#12008=ORIENTED_EDGE ( 'NONE', *, *, #12447, .F. ) ;
#12017=VERTEX_POINT ( 'NONE', #12025 ) ;
#12022=DIRECTION ( 'NONE',  ( 0.9960067511297463483, -0.08927794634716618161, 4.818676322152979407E-17 ) ) ;
#12025=CARTESIAN_POINT ( 'NONE',  ( 53.63671053572210923, -2.048907369402450218, -2.499999999999998224 ) ) ;
#12029=ORIENTED_EDGE ( 'NONE', *, *, #9363, .F. ) ;
#12033=CARTESIAN_POINT ( 'NONE',  ( 47.16901142695026294, 17.29003067336574517, -2.499999999999993783 ) ) ;
#12035=ORIENTED_EDGE ( 'NONE', *, *, #6195, .T. ) ;
#12044=ORIENTED_EDGE ( 'NONE', *, *, #10660, .T. ) ;
#12045=ORIENTED_EDGE ( 'NONE', *, *, #11583, .F. ) ;
#12047=EDGE_LOOP ( 'NONE', ( #2628, #5118, #10333, #8789 ) ) ;
#12048=CARTESIAN_POINT ( 'NONE',  ( 35.65577094119244350, -20.24578327824959345, -2.500000000000003997 ) ) ;
#12054=CARTESIAN_POINT ( 'NONE',  ( 14.53672965213156942, 15.21527412409548674, 3.469446951953614189E-15 ) ) ;
#12056=CARTESIAN_POINT ( 'NONE',  ( 9.857979974958242408, 4.257796268226282876, -2.499999999999999112 ) ) ;
#12065=CIRCLE ( 'NONE', #6475, 9.000000000008999024 ) ;
#12066=DIRECTION ( 'NONE',  ( -0.8735848310779960046, 0.4866719047884613403, 6.939263997980181797E-17 ) ) ;
#12072=DIRECTION ( 'NONE',  ( 0.9960067511297464593, -0.08927794634716622324, 3.401418580343279473E-17 ) ) ;
#12077=DIRECTION ( 'NONE',  ( 0.9960067511297464593, -0.08927794634716622324, 6.802837160686558945E-17 ) ) ;
#12080=ADVANCED_FACE ( 'NONE', ( #10756 ), #127, .T. ) ;
#12083=CARTESIAN_POINT ( 'NONE',  ( 17.19653809941365452, 5.878923826270380459, 2.500000000000000444 ) ) ;
#12090=ADVANCED_FACE ( 'NONE', ( #7812 ), #4814, .T. ) ;
#12091=DIRECTION ( 'NONE',  ( 0.4206864060305147146, -0.9072061219927526343, -2.313087999326727677E-16 ) ) ;
#12105=AXIS2_PLACEMENT_3D ( 'NONE', #10199, #5859, #9080 ) ;
#12110=DIRECTION ( 'NONE',  ( 0.9063077870366492705, 0.4226182617407009956, 0.000000000000000000 ) ) ;
#12111=AXIS2_PLACEMENT_3D ( 'NONE', #2871, #7212, #11563 ) ;
#12114=LINE ( 'NONE', #3620, #12661 ) ;
#12126=AXIS2_PLACEMENT_3D ( 'NONE', #3180, #6414, #7190 ) ;
#12128=EDGE_CURVE ( 'NONE', #2483, #3335, #829, .T. ) ;
#12134=AXIS2_PLACEMENT_3D ( 'NONE', #4270, #13193, #3540 ) ;
#12141=CIRCLE ( 'NONE', #6106, 2.500000000000000444 ) ;
#12147=CARTESIAN_POINT ( 'NONE',  ( 27.98552063842490867, -17.38741154648219833, -2.500000000000004441 ) ) ;
#12151=DIRECTION ( 'NONE',  ( -6.158143864569485777E-17, -2.736152283717910599E-16, 1.000000000000000000 ) ) ;
#12155=ORIENTED_EDGE ( 'NONE', *, *, #6984, .F. ) ;
#12159=DIRECTION ( 'NONE',  ( -6.158143864569485777E-17, -2.736152283717910599E-16, 1.000000000000000000 ) ) ;
#12160=CARTESIAN_POINT ( 'NONE',  ( 34.66997162884352690, 21.14050806081579736, -2.499999999999992895 ) ) ;
#12165=CARTESIAN_POINT ( 'NONE',  ( 10.00024727050385920, -5.026167870790866132, 2.499999999999996891 ) ) ;
#12170=ADVANCED_FACE ( 'NONE', ( #1723, #11265 ), #1582, .T. ) ;
#12177=DIRECTION ( 'NONE',  ( -0.9961946980917455452, -0.08715574274765884588, 0.000000000000000000 ) ) ;
#12187=ADVANCED_FACE ( 'NONE', ( #4877 ), #9154, .T. ) ;
#12194=VECTOR ( 'NONE', #720, 1000.000000000000000 ) ;
#12195=ORIENTED_EDGE ( 'NONE', *, *, #6531, .T. ) ;
#12200=AXIS2_PLACEMENT_3D ( 'NONE', #5176, #3069, #7335 ) ;
#12204=AXIS2_PLACEMENT_3D ( 'NONE', #13821, #8385, #11544 ) ;
#12212=VERTEX_POINT ( 'NONE', #12807 ) ;
#12215=CIRCLE ( 'NONE', #10629, 9.000000000009000800 ) ;
#12216=AXIS2_PLACEMENT_3D ( 'NONE', #4167, #403, #9013 ) ;
#12224=DIRECTION ( 'NONE',  ( 0.9960067511297463483, -0.08927794634716620936, 4.626175998653454121E-17 ) ) ;
#12230=FACE_OUTER_BOUND ( 'NONE', #1548, .T. ) ;
#12239=DIRECTION ( 'NONE',  ( -0.9462100554738961389, -0.3235529800822216639, -1.445602896645893329E-16 ) ) ;
#12244=DIRECTION ( 'NONE',  ( -0.7328050451781165098, -0.6804386568688601811, -2.409338161076489210E-16 ) ) ;
#12257=ORIENTED_EDGE ( 'NONE', *, *, #2888, .T. ) ;
#12269=VERTEX_POINT ( 'NONE', #10349 ) ;
#12271=EDGE_CURVE ( 'NONE', #9210, #3082, #3208, .T. ) ;
#12280=ORIENTED_EDGE ( 'NONE', *, *, #6515, .T. ) ;
#12282=ORIENTED_EDGE ( 'NONE', *, *, #4629, .F. ) ;
#12284=AXIS2_PLACEMENT_3D ( 'NONE', #6819, #1556, #5846 ) ;
#12299=AXIS2_PLACEMENT_3D ( 'NONE', #1945, #9515, #9245 ) ;
#12305=DIRECTION ( 'NONE',  ( -6.158143864569485777E-17, -2.736152283717910599E-16, 1.000000000000000000 ) ) ;
#12307=CARTESIAN_POINT ( 'NONE',  ( 42.70768697973989703, 17.09141780026012469, 2.500000000000005329 ) ) ;
#12310=DIRECTION ( 'NONE',  ( -6.158143864569485777E-17, -2.736152283717910599E-16, 1.000000000000000000 ) ) ;
#12318=SHAPE_REPRESENTATION ( 'Dual Pivoting Lever Wings (x2)', ( #8193 ), #5278 ) ;
#12331=STYLED_ITEM ( 'NONE', ( #8550 ), #7695 ) ;
#12342=AXIS2_PLACEMENT_3D ( 'NONE', #13611, #1581, #2635 ) ;
#12345=AXIS2_PLACEMENT_3D ( 'NONE', #5999, #2771, #12239 ) ;
#12365=VECTOR ( 'NONE', #3437, 1000.000000000000000 ) ;
#12370=EDGE_CURVE ( 'NONE', #12738, #7744, #3419, .T. ) ;
#12373=VERTEX_POINT ( 'NONE', #175 ) ;
#12383=CYLINDRICAL_SURFACE ( 'NONE', #11091, 9.000000000008999024 ) ;
#12384=DIRECTION ( 'NONE',  ( -0.9960067511297463483, 0.08927794634716618161, -4.818676322152979407E-17 ) ) ;
#12385=VERTEX_POINT ( 'NONE', #6669 ) ;
#12390=FACE_OUTER_BOUND ( 'NONE', #11156, .T. ) ;
#12398=AXIS2_PLACEMENT_3D ( 'NONE', #10004, #13184, #3531 ) ;
#12399=ORIENTED_EDGE ( 'NONE', *, *, #7567, .F. ) ;
#12400=VERTEX_POINT ( 'NONE', #3304 ) ;
#12414=DIRECTION ( 'NONE',  ( -6.158143864569485777E-17, -2.736152283717910599E-16, 1.000000000000000000 ) ) ;
#12419=DIRECTION ( 'NONE',  ( 6.158143864569485777E-17, 2.736152283717910599E-16, -1.000000000000000000 ) ) ;
#12436=ORIENTED_EDGE ( 'NONE', *, *, #1642, .T. ) ;
#12438=CIRCLE ( 'NONE', #9739, 9.000000000008999024 ) ;
#12443=CARTESIAN_POINT ( 'NONE',  ( 82.09155748149851206, -71.43674177705591433, 2.500000000000000000 ) ) ;
#12447=EDGE_CURVE ( 'NONE', #10453, #420, #8803, .T. ) ;
#12449=CARTESIAN_POINT ( 'NONE',  ( 39.71817523509052705, -20.60992048131556942, -2.500000000000004441 ) ) ;
#12452=EDGE_CURVE ( 'NONE', #182, #11079, #10600, .T. ) ;
#12454=VECTOR ( 'NONE', #222, 1000.000000000000000 ) ;
#12455=EDGE_CURVE ( 'NONE', #9666, #10021, #8640, .T. ) ;
#12483=EDGE_CURVE ( 'NONE', #12017, #8021, #3664, .T. ) ;
#12484=AXIS2_PLACEMENT_3D ( 'NONE', #6983, #11263, #8950 ) ;
#12486=FACE_OUTER_BOUND ( 'NONE', #2192, .T. ) ;
#12491=ORIENTED_EDGE ( 'NONE', *, *, #13534, .T. ) ;
#12499=DIRECTION ( 'NONE',  ( 0.9960067511297463483, -0.08927794634716618161, 4.818676322152979407E-17 ) ) ;
#12502=CYLINDRICAL_SURFACE ( 'NONE', #7427, 25.50000000002549783 ) ;
#12503=DIRECTION ( 'NONE',  ( -0.08715574274765883200, 0.9961946980917454342, 0.000000000000000000 ) ) ;
#12505=CIRCLE ( 'NONE', #11370, 9.000000000008999024 ) ;
#12509=ORIENTED_EDGE ( 'NONE', *, *, #101, .T. ) ;
#12511=ORIENTED_EDGE ( 'NONE', *, *, #12722, .F. ) ;
#12514=AXIS2_PLACEMENT_3D ( 'NONE', #1393, #363, #12922 ) ;
#12523=DIRECTION ( 'NONE',  ( 0.9960067511297463483, -0.08927794634716618161, 4.818676322152979407E-17 ) ) ;
#12524=AXIS2_PLACEMENT_3D ( 'NONE', #1470, #7850, #2524 ) ;
#12529=ADVANCED_FACE ( 'NONE', ( #12230 ), #658, .T. ) ;
#12535=EDGE_CURVE ( 'NONE', #2174, #3082, #4927, .T. ) ;
#12549=EDGE_CURVE ( 'NONE', #11452, #425, #2544, .T. ) ;
#12551=ORIENTED_EDGE ( 'NONE', *, *, #8748, .T. ) ;
#12563=CYLINDRICAL_SURFACE ( 'NONE', #12111, 9.000000000008999024 ) ;
#12566=CARTESIAN_POINT ( 'NONE',  ( 10.00024727050385920, -5.026167870790865244, -2.500000000000001776 ) ) ;
#12582=CIRCLE ( 'NONE', #4493, 9.000000000008999024 ) ;
#12586=DIRECTION ( 'NONE',  ( -6.158143864569485777E-17, -2.736152283717910599E-16, 1.000000000000000000 ) ) ;
#12598=CARTESIAN_POINT ( 'NONE',  ( 43.29712336220986657, 19.44704974301885159, 2.500000000000005773 ) ) ;
#12608=ORIENTED_EDGE ( 'NONE', *, *, #5147, .T. ) ;
#12614=ADVANCED_FACE ( 'NONE', ( #6255 ), #13731, .T. ) ;
#12617=DIRECTION ( 'NONE',  ( 0.9960067511297463483, -0.08927794634716618161, 4.818676322152979407E-17 ) ) ;
#12624=CIRCLE ( 'NONE', #6563, 9.000000000008999024 ) ;
#12628=EDGE_CURVE ( 'NONE', #7723, #13532, #13389, .T. ) ;
#12637=CYLINDRICAL_SURFACE ( 'NONE', #706, 9.000000000008999024 ) ;
#12639=ORIENTED_EDGE ( 'NONE', *, *, #3442, .T. ) ;
#12646=DIRECTION ( 'NONE',  ( 0.9960067511297463483, -0.08927794634716618161, 4.818676322152979407E-17 ) ) ;
#12654=ORIENTED_EDGE ( 'NONE', *, *, #11067, .F. ) ;
#12655=ORIENTED_EDGE ( 'NONE', *, *, #3780, .T. ) ;
#12657=DIRECTION ( 'NONE',  ( 0.9960067511297464593, -0.08927794634716622324, 3.401418580343279473E-17 ) ) ;
#12661=VECTOR ( 'NONE', #1247, 1000.000000000000000 ) ;
#12662=FACE_OUTER_BOUND ( 'NONE', #321, .T. ) ;
#12665=CYLINDRICAL_SURFACE ( 'NONE', #1568, 2.500000000000000444 ) ;
#12671=ORIENTED_EDGE ( 'NONE', *, *, #1463, .T. ) ;
#12679=CARTESIAN_POINT ( 'NONE',  ( 32.61455173758670867, 25.38817907193537593, 7.372574772901430151E-15 ) ) ;
#12687=ORIENTED_EDGE ( 'NONE', *, *, #11261, .T. ) ;
#12690=ORIENTED_EDGE ( 'NONE', *, *, #12735, .T. ) ;
#12697=EDGE_CURVE ( 'NONE', #2174, #13136, #11763, .T. ) ;
#12705=ORIENTED_EDGE ( 'NONE', *, *, #1118, .F. ) ;
#12713=CYLINDRICAL_SURFACE ( 'NONE', #11556, 18.74900000001875000 ) ;
#12719=CARTESIAN_POINT ( 'NONE',  ( 62.16766351966359849, -73.17985663200910551, 2.500000000000000000 ) ) ;
#12722=EDGE_CURVE ( 'NONE', #11569, #12930, #7721, .T. ) ;
#12735=EDGE_CURVE ( 'NONE', #3156, #7206, #10330, .T. ) ;
#12738=VERTEX_POINT ( 'NONE', #13658 ) ;
#12744=LINE ( 'NONE', #9453, #7174 ) ;
#12748=CARTESIAN_POINT ( 'NONE',  ( 30.29366116764611760, 20.61262658154624816, -2.499999999999993783 ) ) ;
#12777=DIRECTION ( 'NONE',  ( -6.158143864569485777E-17, -2.736152283717910599E-16, 1.000000000000000000 ) ) ;
#12784=CARTESIAN_POINT ( 'NONE',  ( 13.76342357120274862, 14.11587126553561689, 2.500000000000002665 ) ) ;
#12787=AXIS2_PLACEMENT_3D ( 'NONE', #10726, #6535, #12066 ) ;
#12789=CARTESIAN_POINT ( 'NONE',  ( 10.11726280447958182, 5.576682675210008711, 2.500000000000000000 ) ) ;
#12796=EDGE_CURVE ( 'NONE', #1178, #5471, #2371, .T. ) ;
#12801=ADVANCED_FACE ( 'NONE', ( #1198 ), #160, .T. ) ;
#12807=CARTESIAN_POINT ( 'NONE',  ( 76.84607712649204814, -99.92541302764922762, 2.500000000000000000 ) ) ;
#12816=VERTEX_POINT ( 'NONE', #12989 ) ;
#12817=DIRECTION ( 'NONE',  ( 6.158143864569485777E-17, 2.736152283717910599E-16, -1.000000000000000000 ) ) ;
#12829=DIRECTION ( 'NONE',  ( 0.9960067511297464593, -0.08927794634716622324, 6.802837160686558945E-17 ) ) ;
#12830=DIRECTION ( 'NONE',  ( 0.9960067511297463483, -0.08927794634716618161, 4.818676322152979407E-17 ) ) ;
#12842=ORIENTED_EDGE ( 'NONE', *, *, #12991, .F. ) ;
#12844=CIRCLE ( 'NONE', #6784, 18.74900000001875355 ) ;
#12852=( NAMED_UNIT ( * ) PLANE_ANGLE_UNIT ( ) SI_UNIT ( $, .RADIAN. ) );
#12858=VERTEX_POINT ( 'NONE', #9613 ) ;
#12862=AXIS2_PLACEMENT_3D ( 'NONE', #10861, #9970, #4346 ) ;
#12869=LINE ( 'NONE', #1211, #7817 ) ;
#12878=DIRECTION ( 'NONE',  ( 0.9960067511297464593, -0.08927794634716622324, 3.401418580343279473E-17 ) ) ;
#12882=AXIS2_PLACEMENT_3D ( 'NONE', #4056, #11560, #3131 ) ;
#12889=EDGE_CURVE ( 'NONE', #6792, #3113, #13068, .T. ) ;
#12900=CIRCLE ( 'NONE', #12216, 80.00000000000001421 ) ;
#12901=EDGE_CURVE ( 'NONE', #752, #1178, #5730, .T. ) ;
#12907=CYLINDRICAL_SURFACE ( 'NONE', #4297, 18.74900000001875000 ) ;
#12912=ORIENTED_EDGE ( 'NONE', *, *, #5147, .F. ) ;
#12913=ORIENTED_EDGE ( 'NONE', *, *, #10130, .F. ) ;
#12915=( GEOMETRIC_REPRESENTATION_CONTEXT ( 3 ) GLOBAL_UNCERTAINTY_ASSIGNED_CONTEXT ( ( #13197 ) ) GLOBAL_UNIT_ASSIGNED_CONTEXT ( ( #9657, #11758, #4178 ) ) REPRESENTATION_CONTEXT ( 'NONE', 'WORKASPACE' ) );
#12922=DIRECTION ( 'NONE',  ( 0.9960067511297464593, -0.08927794634716622324, 6.802837160686558945E-17 ) ) ;
#12930=VERTEX_POINT ( 'NONE', #12784 ) ;
#12937=DIRECTION ( 'NONE',  ( -6.158143864569485777E-17, -2.736152283717910599E-16, 1.000000000000000000 ) ) ;
#12949=VERTEX_POINT ( 'NONE', #12056 ) ;
#12954=CYLINDRICAL_SURFACE ( 'NONE', #4028, 9.000000000008999024 ) ;
#12958=CARTESIAN_POINT ( 'NONE',  ( 34.99999999999958789, 1.104930248025249758E-13, -2.499999999999999112 ) ) ;
#12964=VECTOR ( 'NONE', #12414, 1000.000000000000000 ) ;
#12970=CYLINDRICAL_SURFACE ( 'NONE', #8441, 18.74900000001875000 ) ;
#12973=AXIS2_PLACEMENT_3D ( 'NONE', #12748, #4315, #12830 ) ;
#12981=ORIENTED_EDGE ( 'NONE', *, *, #7464, .T. ) ;
#12989=CARTESIAN_POINT ( 'NONE',  ( 16.29599561779310335, 1.298160649189403548, 2.499999999999999112 ) ) ;
#12991=EDGE_CURVE ( 'NONE', #11019, #8296, #2606, .T. ) ;
#12995=AXIS2_PLACEMENT_3D ( 'NONE', #3386, #10752, #1168 ) ;
#12996=LINE ( 'NONE', #3363, #9615 ) ;
#12997=LINE ( 'NONE', #3365, #9861 ) ;
#13004=CYLINDRICAL_SURFACE ( 'NONE', #11178, 18.74900000001875000 ) ;
#13012=DIRECTION ( 'NONE',  ( 0.01532218268402011502, -0.9998826084685129567, -2.891205793291787644E-16 ) ) ;
#13015=ORIENTED_EDGE ( 'NONE', *, *, #2347, .T. ) ;
#13031=DIRECTION ( 'NONE',  ( -6.158143864569485777E-17, -2.736152283717910599E-16, 1.000000000000000000 ) ) ;
#13035=ORIENTED_EDGE ( 'NONE', *, *, #8742, .T. ) ;
#13036=DIRECTION ( 'NONE',  ( -0.9960067511297463483, 0.08927794634716618161, -4.818676322152979407E-17 ) ) ;
#13038=ORIENTED_EDGE ( 'NONE', *, *, #13423, .T. ) ;
#13040=AXIS2_PLACEMENT_3D ( 'NONE', #13152, #3575, #9690 ) ;
#13050=ORIENTED_EDGE ( 'NONE', *, *, #2173, .F. ) ;
#13051=ORIENTED_EDGE ( 'NONE', *, *, #7544, .F. ) ;
#13052=EDGE_CURVE ( 'NONE', #2949, #11754, #3104, .T. ) ;
#13058=CARTESIAN_POINT ( 'NONE',  ( 43.14708730495711819, 24.16350488746833136, -2.499999999999992450 ) ) ;
#13060=ADVANCED_FACE ( 'NONE', ( #3962 ), #8235, .T. ) ;
#13063=CARTESIAN_POINT ( 'NONE',  ( 45.47624229149391084, 15.54906262289183871, -2.499999999999994671 ) ) ;
#13068=LINE ( 'NONE', #3424, #785 ) ;
#13074=CARTESIAN_POINT ( 'NONE',  ( 26.69171018101576465, -19.44228176112429551, -2.500000000000004441 ) ) ;
#13079=CYLINDRICAL_SURFACE ( 'NONE', #130, 9.000000000008999024 ) ;
#13094=VERTEX_POINT ( 'NONE', #3046 ) ;
#13118=EDGE_LOOP ( 'NONE', ( #4719, #136, #6205, #13480 ) ) ;
#13123=AXIS2_PLACEMENT_3D ( 'NONE', #5203, #2382, #8769 ) ;
#13126=AXIS2_PLACEMENT_3D ( 'NONE', #9070, #6820, #12077 ) ;
#13129=FACE_OUTER_BOUND ( 'NONE', #3185, .T. ) ;
#13136=VERTEX_POINT ( 'NONE', #6155 ) ;
#13137=PRODUCT_DEFINITION_FORMATION_WITH_SPECIFIED_SOURCE ( 'ANY', '', #9897, .NOT_KNOWN. ) ;
#13138=ORIENTED_EDGE ( 'NONE', *, *, #5395, .T. ) ;
#13142=ORIENTED_EDGE ( 'NONE', *, *, #6132, .F. ) ;
#13144=CARTESIAN_POINT ( 'NONE',  ( 26.69171018101576465, -19.44228176112429551, 2.499999999999994227 ) ) ;
#13147=AXIS2_PLACEMENT_3D ( 'NONE', #656, #2963, #10395 ) ;
#13152=CARTESIAN_POINT ( 'NONE',  ( 34.99999999999958789, 1.091249486606660213E-13, 2.500000000000000000 ) ) ;
#13160=VERTEX_POINT ( 'NONE', #6015 ) ;
#13164=DIRECTION ( 'NONE',  ( -0.8735848310779960046, 0.4866719047884612293, 9.637352644305955116E-17 ) ) ;
#13166=CYLINDRICAL_SURFACE ( 'NONE', #11888, 18.74900000001875000 ) ;
#13169=ORIENTED_EDGE ( 'NONE', *, *, #2347, .F. ) ;
#13170=ORIENTED_EDGE ( 'NONE', *, *, #3015, .T. ) ;
#13184=DIRECTION ( 'NONE',  ( -6.158143864569485777E-17, -2.736152283717910599E-16, 1.000000000000000000 ) ) ;
#13192=DIRECTION ( 'NONE',  ( 0.9960067511297463483, -0.08927794634716618161, 4.818676322152979407E-17 ) ) ;
#13193=DIRECTION ( 'NONE',  ( -6.158143864569485777E-17, -2.736152283717910599E-16, 1.000000000000000000 ) ) ;
#13195=CARTESIAN_POINT ( 'NONE',  ( 58.40844909094411719, 10.11407490371516182, 4.770489558936219510E-15 ) ) ;
#13197=UNCERTAINTY_MEASURE_WITH_UNIT (LENGTH_MEASURE( 1.000000000000000082E-05 ), #9657, 'distance_accuracy_value', 'NONE');
#13204=ORIENTED_EDGE ( 'NONE', *, *, #3429, .F. ) ;
#13207=CIRCLE ( 'NONE', #6902, 2.500000000000000444 ) ;
#13211=CARTESIAN_POINT ( 'NONE',  ( 89.49979561504950709, -156.1132911148542917, 2.500000000000000000 ) ) ;
#13212=CARTESIAN_POINT ( 'NONE',  ( 34.99999999999958789, 1.104930248025249758E-13, -2.499999999999999112 ) ) ;
#13213=DIRECTION ( 'NONE',  ( 0.9960067511297463483, -0.08927794634716619548, 0.000000000000000000 ) ) ;
#13214=ORIENTED_EDGE ( 'NONE', *, *, #11775, .T. ) ;
#13216=ORIENTED_EDGE ( 'NONE', *, *, #9693, .F. ) ;
#13230=CIRCLE ( 'NONE', #1110, 9.000000000008999024 ) ;
#13241=DIRECTION ( 'NONE',  ( 0.9960067511297463483, -0.08927794634716618161, 4.818676322152979407E-17 ) ) ;
#13246=ORIENTED_EDGE ( 'NONE', *, *, #9523, .F. ) ;
#13258=DIRECTION ( 'NONE',  ( -6.158143864569485777E-17, -2.736152283717910599E-16, 1.000000000000000000 ) ) ;
#13260=AXIS2_PLACEMENT_3D ( 'NONE', #9692, #8701, #2321 ) ;
#13261=DIRECTION ( 'NONE',  ( 0.9960067511297463483, -0.08927794634716618161, 4.818676322152979407E-17 ) ) ;
#13266=CARTESIAN_POINT ( 'NONE',  ( 14.53672965213156942, 15.21527412409548852, -2.499999999999996447 ) ) ;
#13274=VECTOR ( 'NONE', #9669, 1000.000000000000000 ) ;
#13275=AXIS2_PLACEMENT_3D ( 'NONE', #8054, #1311, #10092 ) ;
#13282=ORIENTED_EDGE ( 'NONE', *, *, #6804, .T. ) ;
#13284=LINE ( 'NONE', #1395, #3128 ) ;
#13304=DIRECTION ( 'NONE',  ( 0.9960067511297464593, -0.08927794634716622324, 3.401418580343279473E-17 ) ) ;
#13318=AXIS2_PLACEMENT_3D ( 'NONE', #5644, #13892, #12829 ) ;
#13319=ORIENTED_EDGE ( 'NONE', *, *, #9601, .T. ) ;
#13321=ORIENTED_EDGE ( 'NONE', *, *, #13612, .T. ) ;
#13325=AXIS2_PLACEMENT_3D ( 'NONE', #8859, #3272, #4118 ) ;
#13328=CIRCLE ( 'NONE', #7239, 18.74900000001875000 ) ;
#13343=DIRECTION ( 'NONE',  ( -0.4226182617407009401, 0.9063077870366491595, 0.000000000000000000 ) ) ;
#13353=ADVANCED_FACE ( 'NONE', ( #11608 ), #11807, .T. ) ;
#13358=EDGE_LOOP ( 'NONE', ( #315, #460, #4015, #10929 ) ) ;
#13371=ADVANCED_FACE ( 'NONE', ( #6484 ), #10750, .T. ) ;
#13389=CIRCLE ( 'NONE', #4597, 9.000000000008999024 ) ;
#13401=ORIENTED_EDGE ( 'NONE', *, *, #13870, .F. ) ;
#13406=CARTESIAN_POINT ( 'NONE',  ( 155.9864723944028810, -111.6214737678657087, 2.500000000000000000 ) ) ;
#13423=EDGE_CURVE ( 'NONE', #13532, #13094, #3055, .T. ) ;
#13429=DIRECTION ( 'NONE',  ( -0.9960067511297463483, 0.08927794634716619548, -4.626175998653453504E-17 ) ) ;
#13436=EDGE_CURVE ( 'NONE', #3703, #4205, #12900, .T. ) ;
#13449=AXIS2_PLACEMENT_3D ( 'NONE', #4002, #788, #10457 ) ;
#13454=DIRECTION ( 'NONE',  ( -6.158143864569485777E-17, -2.736152283717910599E-16, 1.000000000000000000 ) ) ;
#13475=DIRECTION ( 'NONE',  ( -0.6001121574638170753, 0.7999158696163758409, 1.927470528861191763E-16 ) ) ;
#13477=DIRECTION ( 'NONE',  ( 0.9960067511297463483, -0.08927794634716618161, 4.818676322152979407E-17 ) ) ;
#13479=CARTESIAN_POINT ( 'NONE',  ( 62.16766351966359849, -73.17985663200910551, 2.500000000000000000 ) ) ;
#13480=ORIENTED_EDGE ( 'NONE', *, *, #13436, .T. ) ;
#13485=VERTEX_POINT ( 'NONE', #12165 ) ;
#13492=CARTESIAN_POINT ( 'NONE',  ( 55.20422767451771051, -6.230504303137470501, -2.499999999999999112 ) ) ;
#13493=DIRECTION ( 'NONE',  ( -6.158143864569485777E-17, -2.736152283717910599E-16, 1.000000000000000000 ) ) ;
#13496=VECTOR ( 'NONE', #8836, 1000.000000000000000 ) ;
#13499=EDGE_CURVE ( 'NONE', #4205, #9863, #6839, .T. ) ;
#13504=ORIENTED_EDGE ( 'NONE', *, *, #8325, .T. ) ;
#13510=CIRCLE ( 'NONE', #9215, 25.50000000002549783 ) ;
#13522=DIRECTION ( 'NONE',  ( 6.158143864569485777E-17, 2.736152283717910599E-16, -1.000000000000000000 ) ) ;
#13525=CIRCLE ( 'NONE', #11454, 18.74900000001875355 ) ;
#13532=VERTEX_POINT ( 'NONE', #9778 ) ;
#13534=EDGE_CURVE ( 'NONE', #7120, #11569, #12438, .T. ) ;
#13545=DIRECTION ( 'NONE',  ( -1.000000000000000000, 0.000000000000000000, 0.000000000000000000 ) ) ;
#13557=DIRECTION ( 'NONE',  ( 0.9960067511297463483, -0.08927794634716618161, 4.818676322152979407E-17 ) ) ;
#13562=AXIS2_PLACEMENT_3D ( 'NONE', #3376, #1157, #5413 ) ;
#13564=ORIENTED_EDGE ( 'NONE', *, *, #12697, .T. ) ;
#13572=LINE ( 'NONE', #2874, #864 ) ;
#13584=DIRECTION ( 'NONE',  ( -6.158143864569485777E-17, -2.736152283717910599E-16, 1.000000000000000000 ) ) ;
#13605=DIRECTION ( 'NONE',  ( 0.4206864060305147146, -0.9072061219927525233, -2.409338161076489703E-16 ) ) ;
#13611=CARTESIAN_POINT ( 'NONE',  ( 55.00383357371546822, 6.846651893462918359, 2.500000000000003109 ) ) ;
#13612=EDGE_CURVE ( 'NONE', #3335, #6530, #2773, .T. ) ;
#13617=ORIENTED_EDGE ( 'NONE', *, *, #5963, .T. ) ;
#13622=ORIENTED_EDGE ( 'NONE', *, *, #10066, .F. ) ;
#13634=ORIENTED_EDGE ( 'NONE', *, *, #4816, .T. ) ;
#13637=CARTESIAN_POINT ( 'NONE',  ( 80.29381926039658879, -64.72749139719506672, 2.500000000000000000 ) ) ;
#13638=CARTESIAN_POINT ( 'NONE',  ( 52.82363224725100537, -5.817485239812894449, 2.500000000000000000 ) ) ;
#13645=ORIENTED_EDGE ( 'NONE', *, *, #10963, .T. ) ;
#13658=CARTESIAN_POINT ( 'NONE',  ( 32.50998312217522113, 0.2231948658680255881, -2.499999999999997335 ) ) ;
#13690=ORIENTED_EDGE ( 'NONE', *, *, #12128, .T. ) ;
#13697=CARTESIAN_POINT ( 'NONE',  ( 82.09155748149851206, -71.43674177705591433, 2.500000000000000000 ) ) ;
#13702=AXIS2_PLACEMENT_3D ( 'NONE', #1019, #10549, #2914 ) ;
#13707=CARTESIAN_POINT ( 'NONE',  ( 53.56517978609545594, 2.618988451796029349, -2.499999999999997335 ) ) ;
#13709=CIRCLE ( 'NONE', #9656, 20.00000000000001066 ) ;
#13712=LINE ( 'NONE', #10503, #10102 ) ;
#13718=CIRCLE ( 'NONE', #5167, 9.000000000008999024 ) ;
#13723=ORIENTED_EDGE ( 'NONE', *, *, #8748, .F. ) ;
#13724=DIRECTION ( 'NONE',  ( -6.158143864569485777E-17, -2.736152283717910599E-16, 1.000000000000000000 ) ) ;
#13731=CYLINDRICAL_SURFACE ( 'NONE', #5967, 25.50000000002549783 ) ;
#13732=ORIENTED_EDGE ( 'NONE', *, *, #10660, .F. ) ;
#13733=ORIENTED_EDGE ( 'NONE', *, *, #7997, .T. ) ;
#13734=ORIENTED_EDGE ( 'NONE', *, *, #2309, .F. ) ;
#13744=DIRECTION ( 'NONE',  ( -6.158143864569485777E-17, -2.736152283717910599E-16, 1.000000000000000000 ) ) ;
#13745=DIRECTION ( 'NONE',  ( -6.158143864569485777E-17, -2.736152283717910599E-16, 1.000000000000000000 ) ) ;
#13748=FACE_OUTER_BOUND ( 'NONE', #1999, .T. ) ;
#13759=DIRECTION ( 'NONE',  ( -6.158143864569485777E-17, -2.736152283717910599E-16, 1.000000000000000000 ) ) ;
#13761=EDGE_CURVE ( 'NONE', #3156, #13094, #4133, .T. ) ;
#13763=CYLINDRICAL_SURFACE ( 'NONE', #12299, 80.00000000000001421 ) ;
#13769=CIRCLE ( 'NONE', #1645, 9.000000000009002576 ) ;
#13770=DIRECTION ( 'NONE',  ( 6.158143864569485777E-17, 2.736152283717910599E-16, -1.000000000000000000 ) ) ;
#13773=EDGE_CURVE ( 'NONE', #1244, #10453, #3249, .T. ) ;
#13777=ADVANCED_FACE ( 'NONE', ( #8366 ), #7440, .T. ) ;
#13787=CARTESIAN_POINT ( 'NONE',  ( 82.09155748149851206, -71.43674177705591433, -2.500000000000000000 ) ) ;
#13800=VERTEX_POINT ( 'NONE', #10534 ) ;
#13804=DIRECTION ( 'NONE',  ( 6.158143864569485777E-17, 2.736152283717910599E-16, -1.000000000000000000 ) ) ;
#13809=AXIS2_PLACEMENT_3D ( 'NONE', #4102, #6418, #11675 ) ;
#13810=DIRECTION ( 'NONE',  ( -0.8735848310779960046, 0.4866719047884613403, 6.939263997980181797E-17 ) ) ;
#13815=ORIENTED_EDGE ( 'NONE', *, *, #11583, .T. ) ;
#13821=CARTESIAN_POINT ( 'NONE',  ( 34.99999999999958789, 1.091249486606660213E-13, 2.500000000000000000 ) ) ;
#13825=CYLINDRICAL_SURFACE ( 'NONE', #4863, 9.000000000008999024 ) ;
#13828=CYLINDRICAL_SURFACE ( 'NONE', #12973, 9.000000000008999024 ) ;
#13831=EDGE_CURVE ( 'NONE', #11850, #11500, #3100, .T. ) ;
#13833=CIRCLE ( 'NONE', #13147, 9.000000000008999024 ) ;
#13851=DIRECTION ( 'NONE',  ( -6.158143864569485777E-17, -2.736152283717910599E-16, 1.000000000000000000 ) ) ;
#13860=ORIENTED_EDGE ( 'NONE', *, *, #12697, .F. ) ;
#13862=EDGE_LOOP ( 'NONE', ( #9681, #167, #1892, #13170 ) ) ;
#13863=ORIENTED_EDGE ( 'NONE', *, *, #6103, .T. ) ;
#13870=EDGE_CURVE ( 'NONE', #8314, #10021, #9750, .T. ) ;
#13872=DIRECTION ( 'NONE',  ( -0.6001121574638170753, 0.7999158696163758409, 1.850470399461381402E-16 ) ) ;
#13877=CIRCLE ( 'NONE', #8918, 9.000000000008999024 ) ;
#13883=ORIENTED_EDGE ( 'NONE', *, *, #9972, .T. ) ;
#13892=DIRECTION ( 'NONE',  ( -6.158143864569485777E-17, -2.736152283717910599E-16, 1.000000000000000000 ) ) ;
#13893=DIRECTION ( 'NONE',  ( -6.158143864569485777E-17, -2.736152283717910599E-16, 1.000000000000000000 ) ) ;
#13896=FILL_AREA_STYLE_COLOUR ( '', #3720 ) ;
ENDSEC;
END-ISO-10303-21;
